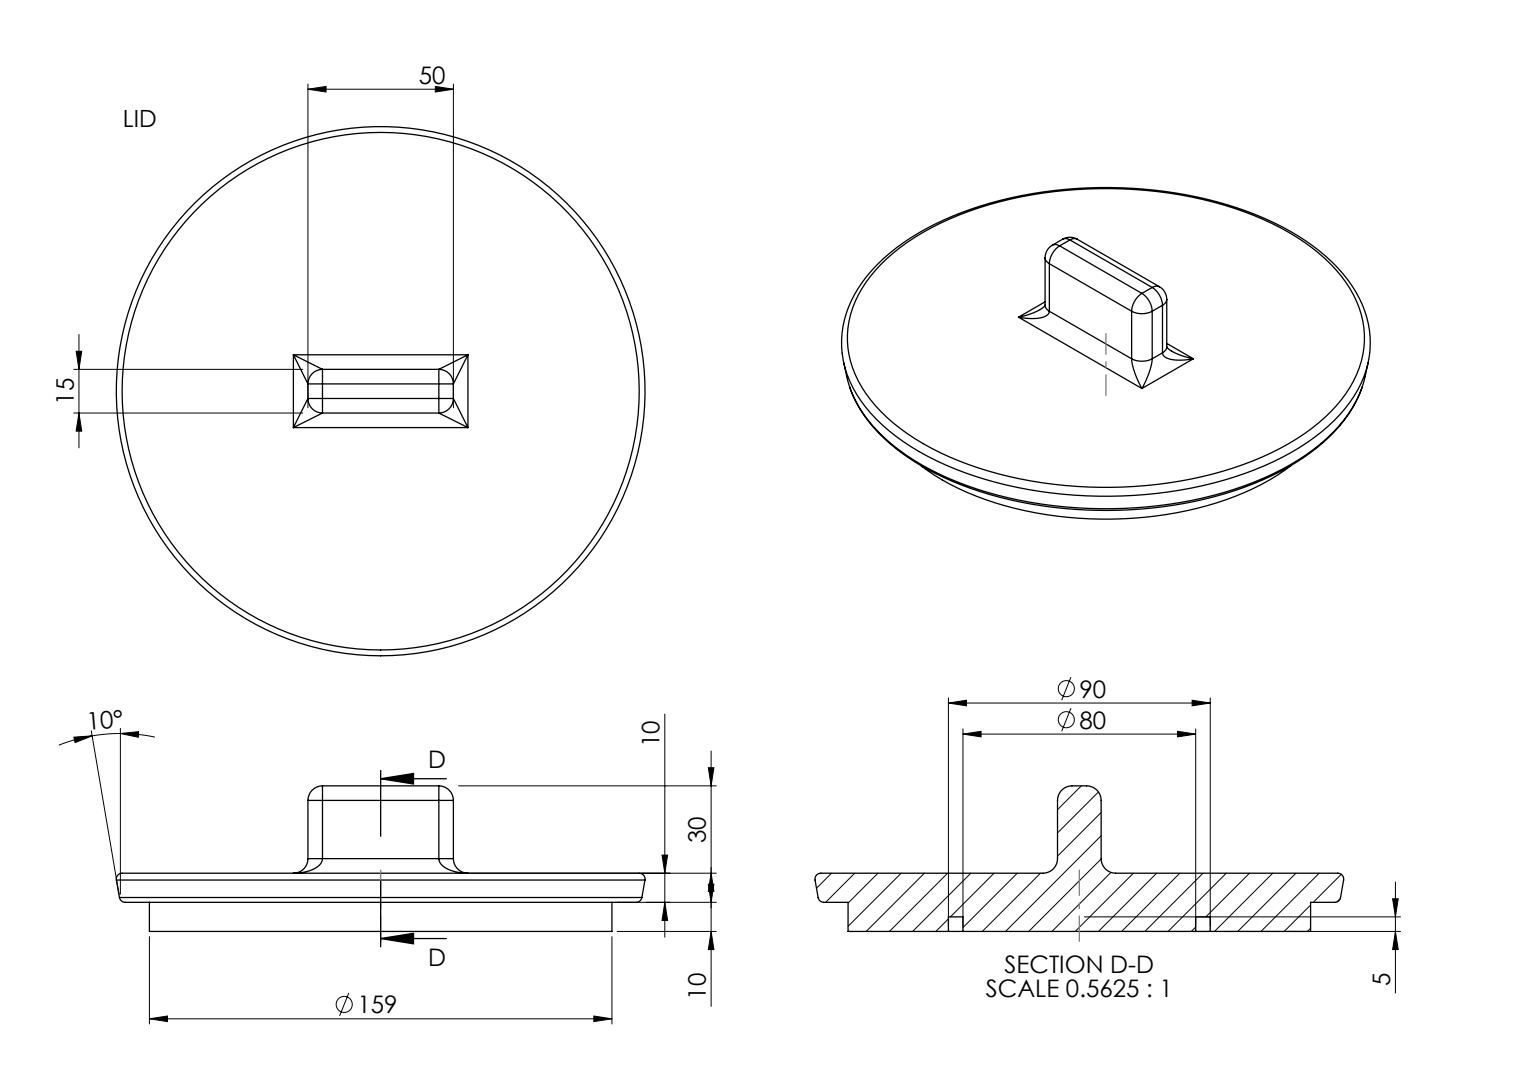
ISO-10303-21;
HEADER;
FILE_DESCRIPTION (('STEP AP214'),
    '1' );
FILE_NAME ('lid.step',
    '2026-10-09T15:02:13',
    ( '' ),
    ( '' ),
    'SwSTEP 2.0',
    'SolidWorks 2026',
    '' );
FILE_SCHEMA (( 'AUTOMOTIVE_DESIGN' ));
ENDSEC;

DATA;
#3=DIRECTION ( 'NONE',  ( 0.000000000000000000, 0.000000000000000000, 1.000000000000000000 ) ) ;
#21=EDGE_LOOP ( 'NONE', ( #2044, #4544 ) ) ;
#25=CARTESIAN_POINT ( 'NONE',  ( 21.01167039530690062, 284.7842439685853719, -8.005835197659997959 ) ) ;
#29=EDGE_CURVE ( 'NONE', #8003, #7684, #9198, .T. ) ;
#39=ORIENTED_EDGE ( 'NONE', *, *, #2245, .T. ) ;
#51=CARTESIAN_POINT ( 'NONE',  ( -30.00000000000000711, 282.0000000000000000, 0.000000000000000000 ) ) ;
#52=ORIENTED_EDGE ( 'NONE', *, *, #15437, .T. ) ;
#55=ORIENTED_EDGE ( 'NONE', *, *, #4586, .T. ) ;
#81=VERTEX_POINT ( 'NONE', #16451 ) ;
#88=CARTESIAN_POINT ( 'NONE',  ( 25.00000000000000000, 284.0710678118655323, -2.499999999999998224 ) ) ;
#98=ORIENTED_EDGE ( 'NONE', *, *, #10995, .T. ) ;
#103=CARTESIAN_POINT ( 'NONE',  ( 28.07127062163609210, 282.3184422169448453, -10.57127062163368691 ) ) ;
#134=AXIS2_PLACEMENT_3D ( 'NONE', #8238, #4509, #8316 ) ;
#139=ORIENTED_EDGE ( 'NONE', *, *, #8040, .T. ) ;
#167=AXIS2_PLACEMENT_3D ( 'NONE', #3146, #15868, #1731 ) ;
#168=AXIS2_PLACEMENT_3D ( 'NONE', #2091, #15059, #8742 ) ;
#190=CARTESIAN_POINT ( 'NONE',  ( 24.98849325795415766, 282.6608420050619088, -9.994246628976295455 ) ) ;
#199=EDGE_CURVE ( 'NONE', #14735, #10689, #4239, .T. ) ;
#223=DIRECTION ( 'NONE',  ( 0.000000000000000000, -1.000000000000000000, 0.000000000000000000 ) ) ;
#233=AXIS2_PLACEMENT_3D ( 'NONE', #3422, #4672, #16139 ) ;
#242=LINE ( 'NONE', #9147, #15465 ) ;
#265=UNCERTAINTY_MEASURE_WITH_UNIT (LENGTH_MEASURE( 1.000000000000000082E-05 ), #1967, 'distance_accuracy_value', 'NONE');
#270=CARTESIAN_POINT ( 'NONE',  ( 26.95005104082769876, 283.0244618719127629, -6.400102081653807673 ) ) ;
#274=CARTESIAN_POINT ( 'NONE',  ( -29.67274705320269135, 282.0000000000000000, 11.84549410641580813 ) ) ;
#302=ORIENTED_EDGE ( 'NONE', *, *, #6524, .T. ) ;
#329=SHAPE_REPRESENTATION ( 'lid', ( #15812 ), #9193 ) ;
#349=ORIENTED_EDGE ( 'NONE', *, *, #7162, .F. ) ;
#353=CARTESIAN_POINT ( 'NONE',  ( 20.51073895446616291, 285.3889217077638705, 7.755369477227151975 ) ) ;
#354=CARTESIAN_POINT ( 'NONE',  ( -27.49424662897630256, 282.6608420050619088, 7.488493257954157656 ) ) ;
#368=CARTESIAN_POINT ( 'NONE',  ( 1.100495818310455813E-14, 282.0000000000000000, -88.87749532708107836 ) ) ;
#381=EDGE_LOOP ( 'NONE', ( #515, #9607 ) ) ;
#395=LINE ( 'NONE', #4248, #7805 ) ;
#429=CIRCLE ( 'NONE', #8137, 79.49773270518484480 ) ;
#443=CARTESIAN_POINT ( 'NONE',  ( -30.00000000000000711, 282.0000000000000000, 12.50000000000000000 ) ) ;
#451=AXIS2_PLACEMENT_3D ( 'NONE', #16347, #7624, #4984 ) ;
#464=PRODUCT_CONTEXT ( 'NONE', #15229, 'mechanical' ) ;
#466=DIRECTION ( 'NONE',  ( 0.000000000000000000, 0.000000000000000000, -1.000000000000000000 ) ) ;
#512=EDGE_CURVE ( 'NONE', #3799, #13515, #6038, .T. ) ;
#515=ORIENTED_EDGE ( 'NONE', *, *, #6228, .F. ) ;
#520=CARTESIAN_POINT ( 'NONE',  ( 22.04892374372132835, 283.9500510409123422, 8.524461871856116701 ) ) ;
#521=CARTESIAN_POINT ( 'NONE',  ( -29.34550962211183744, 282.0322304394514390, 11.19101924422352212 ) ) ;
#581=FACE_BOUND ( 'NONE', #14554, .T. ) ;
#586=AXIS2_PLACEMENT_3D ( 'NONE', #1715, #3134, #466 ) ;
#593=CARTESIAN_POINT ( 'NONE',  ( 28.07127062163604947, 282.3184422169448453, 10.57127062163685949 ) ) ;
#594=CARTESIAN_POINT ( 'NONE',  ( -27.61612561546114009, 282.5087415087664908, 10.11612561546189681 ) ) ;
#621=DIRECTION ( 'NONE',  ( 0.000000000000000000, 0.000000000000000000, 1.000000000000000000 ) ) ;
#630=ADVANCED_FACE ( 'NONE', ( #6188 ), #1425, .F. ) ;
#645=ORIENTED_EDGE ( 'NONE', *, *, #4809, .T. ) ;
#653=DIRECTION ( 'NONE',  ( 0.000000000000000000, 1.000000000000000000, 0.000000000000000000 ) ) ;
#656=AXIS2_PLACEMENT_3D ( 'NONE', #7217, #7053, #1959 ) ;
#675=LINE ( 'NONE', #11094, #3539 ) ;
#676=DIRECTION ( 'NONE',  ( 0.000000000000000000, 0.000000000000000000, -1.000000000000000000 ) ) ;
#714=EDGE_LOOP ( 'NONE', ( #14088, #8765 ) ) ;
#721=CARTESIAN_POINT ( 'NONE',  ( 0.000000000000000000, 272.0000000000000000, 0.000000000000000000 ) ) ;
#728=CARTESIAN_POINT ( 'NONE',  ( 0.000000000000000000, 282.0000000000000000, 0.000000000000000000 ) ) ;
#750=DIRECTION ( 'NONE',  ( 0.000000000000000000, 1.000000000000000000, 0.000000000000000000 ) ) ;
#785=ADVANCED_FACE ( 'NONE', ( #11984 ), #5440, .T. ) ;
#827=DIRECTION ( 'NONE',  ( 1.734723475976807094E-17, 0.000000000000000000, -1.000000000000000000 ) ) ;
#832=EDGE_CURVE ( 'NONE', #2646, #12589, #15834, .T. ) ;
#846=ADVANCED_FACE ( 'NONE', ( #581, #11664 ), #5365, .T. ) ;
#862=ORIENTED_EDGE ( 'NONE', *, *, #15437, .F. ) ;
#870=CARTESIAN_POINT ( 'NONE',  ( -26.23306594130729863, 283.6958662468272792, -4.966131882590582691 ) ) ;
#872=TOROIDAL_SURFACE ( 'NONE', #3283, 88.87749532708107836, 2.000000000000000000 ) ;
#881=LINE ( 'NONE', #9625, #1539 ) ;
#887=CARTESIAN_POINT ( 'NONE',  ( 30.00000000000000000, 282.0000000000000000, 12.50000000000000178 ) ) ;
#891=VERTEX_POINT ( 'NONE', #12993 ) ;
#902=CARTESIAN_POINT ( 'NONE',  ( -2.168404344971008868E-16, 282.0000000000000000, 12.50000000000000000 ) ) ;
#909=CARTESIAN_POINT ( 'NONE',  ( 0.000000000000000000, 262.0000000000000000, 79.49773270518484480 ) ) ;
#944=CARTESIAN_POINT ( 'NONE',  ( 0.000000000000000000, 262.0000000000000000, 0.000000000000000000 ) ) ;
#952=CARTESIAN_POINT ( 'NONE',  ( -24.93825083352641769, 285.3724546740604637, -7.438250833528329942 ) ) ;
#1003=CARTESIAN_POINT ( 'NONE',  ( -25.00000000000000711, 284.0710678118655323, -2.499999999999999556 ) ) ;
#1004=EDGE_LOOP ( 'NONE', ( #10265, #9223, #9244, #3240 ) ) ;
#1036=CARTESIAN_POINT ( 'NONE',  ( -26.95005104082770231, 283.0244618719127629, -6.400102081653810338 ) ) ;
#1039=FACE_OUTER_BOUND ( 'NONE', #9562, .T. ) ;
#1042=VERTEX_POINT ( 'NONE', #14706 ) ;
#1043=DIRECTION ( 'NONE',  ( 0.000000000000000000, 0.000000000000000000, 1.000000000000000000 ) ) ;
#1051=SURFACE_STYLE_USAGE ( .BOTH. , #4992 ) ;
#1066=ORIENTED_EDGE ( 'NONE', *, *, #4920, .T. ) ;
#1070=LINE ( 'NONE', #6161, #12897 ) ;
#1073=DIRECTION ( 'NONE',  ( 0.000000000000000000, 0.000000000000000000, 1.000000000000000000 ) ) ;
#1075=DIRECTION ( 'NONE',  ( -0.000000000000000000, -1.000000000000000000, -0.000000000000000000 ) ) ;
#1106=FACE_OUTER_BOUND ( 'NONE', #13659, .T. ) ;
#1114=CARTESIAN_POINT ( 'NONE',  ( -24.96465690379244862, 286.9981936728224241, -7.464656903793316367 ) ) ;
#1122=CARTESIAN_POINT ( 'NONE',  ( 19.99999999999999289, 307.0000000000000568, -7.500000000000000000 ) ) ;
#1127=( NAMED_UNIT ( * ) SI_UNIT ( $, .STERADIAN. ) SOLID_ANGLE_UNIT ( ) );
#1149=CARTESIAN_POINT ( 'NONE',  ( 25.00000000000000000, 284.0710678118655323, 2.500000000000002220 ) ) ;
#1154=( BOUNDED_CURVE ( )  B_SPLINE_CURVE ( 3, ( #10835, #1003, #11172, #4860 ),
 .UNSPECIFIED., .F., .F. ) 
 B_SPLINE_CURVE_WITH_KNOTS ( ( 4, 4 ),
 ( 3.141592653589793116, 4.712388980384689674 ),
 .UNSPECIFIED. ) 
 CURVE ( )  GEOMETRIC_REPRESENTATION_ITEM ( )  RATIONAL_B_SPLINE_CURVE ( ( 1.000000000000000000, 0.8047378541243649375, 0.8047378541243649375, 1.000000000000000000 ) ) 
 REPRESENTATION_ITEM ( '' )  );
#1171=CARTESIAN_POINT ( 'NONE',  ( 27.07106781186548261, 282.0000000000000000, -6.642135623730952787 ) ) ;
#1184=ORIENTED_EDGE ( 'NONE', *, *, #14174, .T. ) ;
#1197=CARTESIAN_POINT ( 'NONE',  ( -24.86904120090709469, 286.8604097559688739, -7.369041200906229605 ) ) ;
#1209=FACE_OUTER_BOUND ( 'NONE', #12628, .T. ) ;
#1214=EDGE_CURVE ( 'NONE', #8474, #14735, #13959, .T. ) ;
#1223=ORIENTED_EDGE ( 'NONE', *, *, #1722, .F. ) ;
#1226=VERTEX_POINT ( 'NONE', #7814 ) ;
#1247=AXIS2_PLACEMENT_3D ( 'NONE', #12774, #6216, #11211 ) ;
#1255=AXIS2_PLACEMENT_3D ( 'NONE', #8224, #5420, #13290 ) ;
#1277=CARTESIAN_POINT ( 'NONE',  ( 25.50583519765982743, 284.7842439685857698, -3.511670395308112536 ) ) ;
#1303=DIRECTION ( 'NONE',  ( 0.000000000000000000, 0.000000000000000000, 1.000000000000000000 ) ) ;
#1322=DIRECTION ( 'NONE',  ( 0.000000000000000000, -1.000000000000000000, 0.000000000000000000 ) ) ;
#1329=ADVANCED_FACE ( 'NONE', ( #5419 ), #15589, .T. ) ;
#1333=ORIENTED_EDGE ( 'NONE', *, *, #14008, .T. ) ;
#1340=CARTESIAN_POINT ( 'NONE',  ( 25.00000000000000000, 287.0000000000000568, -2.499999999999997780 ) ) ;
#1355=CARTESIAN_POINT ( 'NONE',  ( 23.39173249367926388, 283.2330659412876344, -9.195866246846929215 ) ) ;
#1380=LINE ( 'NONE', #12700, #5056 ) ;
#1402=CARTESIAN_POINT ( 'NONE',  ( 0.000000000000000000, 267.0000000000000000, 0.000000000000000000 ) ) ;
#1409=ORIENTED_EDGE ( 'NONE', *, *, #2371, .T. ) ;
#1410=AXIS2_PLACEMENT_3D ( 'NONE', #16214, #14542, #13953 ) ;
#1417=DIRECTION ( 'NONE',  ( 0.000000000000000000, -1.000000000000000000, 0.000000000000000000 ) ) ;
#1425=CYLINDRICAL_SURFACE ( 'NONE', #14242, 5.000000000000000888 ) ;
#1455=ORIENTED_EDGE ( 'NONE', *, *, #11697, .T. ) ;
#1473=CIRCLE ( 'NONE', #15285, 5.000000000000000000 ) ;
#1486=FACE_OUTER_BOUND ( 'NONE', #4355, .T. ) ;
#1520=CARTESIAN_POINT ( 'NONE',  ( -4.336808689942020818E-17, 307.0000000000000568, 2.500000000000001776 ) ) ;
#1528=CARTESIAN_POINT ( 'NONE',  ( 26.02446187186532001, 283.9500510408986429, -4.548923743720680868 ) ) ;
#1530=DIRECTION ( 'NONE',  ( -1.000000000000000000, -0.000000000000000000, -1.734723475976807094E-17 ) ) ;
#1532=CARTESIAN_POINT ( 'NONE',  ( -26.23306594130729863, 283.6958662468272792, 4.966131882590584468 ) ) ;
#1539=VECTOR ( 'NONE', #7143, 1000.000000000000000 ) ;
#1572=DIRECTION ( 'NONE',  ( 0.000000000000000000, -1.000000000000000000, 0.000000000000000000 ) ) ;
#1580=DIRECTION ( 'NONE',  ( -0.000000000000000000, -1.000000000000000000, -0.000000000000000000 ) ) ;
#1603=( BOUNDED_SURFACE ( )  B_SPLINE_SURFACE ( 3, 2, ( 
 ( #6296, #4813, #7207 ),
 ( #11029, #3384, #2287 ),
 ( #8777, #13760, #10038 ),
 ( #3547, #9866, #14751 ),
 ( #16098, #4732, #7532 ),
 ( #8600, #11365, #8524 ),
 ( #13514, #7379, #12445 ),
 ( #1036, #13839, #12523 ),
 ( #2198, #12268, #7456 ),
 ( #870, #2453, #11204 ),
 ( #7295, #952, #15002 ),
 ( #9790, #11123, #5966 ),
 ( #12603, #12351, #16256 ),
 ( #6053, #4890, #9947 ),
 ( #3638, #1197, #8694 ),
 ( #2373, #1114, #16432 ),
 ( #6210, #11281, #12998 ),
 ( #4101, #11444, #10425 ) ),
 .UNSPECIFIED., .F., .F., .F. ) 
 B_SPLINE_SURFACE_WITH_KNOTS ( ( 4, 2, 2, 2, 2, 2, 2, 2, 4 ),
 ( 3, 3 ),
 ( 1.570796326794896558, 1.767145867644258628, 1.963495408493620697, 2.159844949342982545, 2.356194490192344837, 2.552544031041707129, 2.748893571891068976, 2.945243112740430824, 3.141592653589793116 ),
 ( 0.000000000000000000, 1.000000000000000000 ),
 .UNSPECIFIED. ) 
 GEOMETRIC_REPRESENTATION_ITEM ( )  RATIONAL_B_SPLINE_SURFACE ( (
 ( 1.000000000000000000, 1.000000000000000000, 1.000000000000000000),
 ( 1.000000000000000000, 1.000000000000000000, 1.000000000000000000),
 ( 1.000000000000000000, 0.9967613244521498217, 1.000000000000000000),
 ( 1.000000000000000000, 0.9841171504955907867, 1.000000000000000000),
 ( 1.000000000000000000, 0.9747108043452232806, 1.000000000000000000),
 ( 1.000000000000000000, 0.9506740354170890583, 1.000000000000000000),
 ( 1.000000000000000000, 0.9360421842396997594, 1.000000000000000000),
 ( 1.000000000000000000, 0.9031650994466968729, 1.000000000000000000),
 ( 1.000000000000000000, 0.8849191470854506081, 1.000000000000000000),
 ( 1.000000000000000000, 0.8471316604834270292, 1.000000000000000000),
 ( 1.000000000000000000, 0.8275942695279743244, 1.000000000000000000),
 ( 1.000000000000000000, 0.7902180087153679588, 1.000000000000000000),
 ( 1.000000000000000000, 0.7723968217385259738, 1.000000000000000000),
 ( 1.000000000000000000, 0.7418334179586800747, 1.000000000000000000),
 ( 1.000000000000000000, 0.7291288939600593100, 1.000000000000000000),
 ( 1.000000000000000000, 0.7117460025832584858, 1.000000000000000000),
 ( 1.000000000000000000, 0.7070717283367141670, 1.000000000000000000),
 ( 1.000000000000000000, 0.7071067811865475727, 1.000000000000000000) ) ) 
 REPRESENTATION_ITEM ( '' )  SURFACE ( )  );
#1606=CARTESIAN_POINT ( 'NONE',  ( 21.32168401022778070, 284.4942466289054437, -8.160842005109239850 ) ) ;
#1609=FACE_OUTER_BOUND ( 'NONE', #8042, .T. ) ;
#1610=CARTESIAN_POINT ( 'NONE',  ( -26.77784341583514305, 282.2553694771637538, 10.88892170791705283 ) ) ;
#1613=CARTESIAN_POINT ( 'NONE',  ( 0.000000000000000000, 262.0000000000000000, 0.000000000000000000 ) ) ;
#1689=CARTESIAN_POINT ( 'NONE',  ( 24.96465690379361035, 286.9981936728412393, 7.464656903795364506 ) ) ;
#1691=CARTESIAN_POINT ( 'NONE',  ( -20.31983351293596129, 285.7035871579731179, 7.659916756467385568 ) ) ;
#1715=CARTESIAN_POINT ( 'NONE',  ( 0.000000000000000000, 267.0000000000000000, 0.000000000000000000 ) ) ;
#1722=EDGE_CURVE ( 'NONE', #13617, #14735, #2050, .T. ) ;
#1731=DIRECTION ( 'NONE',  ( 1.224646799147349509E-16, 0.000000000000000000, -1.000000000000000000 ) ) ;
#1748=EDGE_LOOP ( 'NONE', ( #7738, #12625, #11533, #2666 ) ) ;
#1763=AXIS2_PLACEMENT_3D ( 'NONE', #3834, #2583, #12728 ) ;
#1774=CARTESIAN_POINT ( 'NONE',  ( 23.90010208165380590, 283.0244618719131040, 9.450051040827188942 ) ) ;
#1776=CARTESIAN_POINT ( 'NONE',  ( -28.69101924422432148, 282.0322304394514390, 11.84550962211183567 ) ) ;
#1785=AXIS2_PLACEMENT_3D ( 'NONE', #10647, #9394, #14203 ) ;
#1857=EDGE_CURVE ( 'NONE', #3799, #8474, #14802, .T. ) ;
#1923=CARTESIAN_POINT ( 'NONE',  ( 21.32168401022777360, 284.4942466288916307, 8.160842005118437825 ) ) ;
#1933=EDGE_CURVE ( 'NONE', #8272, #81, #7384, .T. ) ;
#1938=ADVANCED_FACE ( 'NONE', ( #16357, #4997 ), #2715, .F. ) ;
#1959=DIRECTION ( 'NONE',  ( 0.000000000000000000, 0.000000000000000000, -1.000000000000000000 ) ) ;
#1967=( LENGTH_UNIT ( ) NAMED_UNIT ( * ) SI_UNIT ( .MILLI., .METRE. ) );
#1985=DIRECTION ( 'NONE',  ( -1.000000000000000000, 0.000000000000000000, -1.734723475976807094E-17 ) ) ;
#2001=AXIS2_PLACEMENT_3D ( 'NONE', #6202, #15242, #4030 ) ;
#2011=CARTESIAN_POINT ( 'NONE',  ( 25.00000000000000000, 287.0000000000000568, 2.500000000000001776 ) ) ;
#2012=CARTESIAN_POINT ( 'NONE',  ( -25.00000000000001066, 287.0000000000000000, 7.500000000000002665 ) ) ;
#2024=EDGE_CURVE ( 'NONE', #10428, #13519, #881, .T. ) ;
#2041=VECTOR ( 'NONE', #1043, 1000.000000000000000 ) ;
#2044=ORIENTED_EDGE ( 'NONE', *, *, #16095, .T. ) ;
#2050=CIRCLE ( 'NONE', #1255, 5.000000000000000000 ) ;
#2052=DIRECTION ( 'NONE',  ( 0.000000000000000000, 1.000000000000000000, 0.000000000000000000 ) ) ;
#2067=ORIENTED_EDGE ( 'NONE', *, *, #5119, .F. ) ;
#2091=CARTESIAN_POINT ( 'NONE',  ( 0.000000000000000000, 267.0000000000000000, 0.000000000000000000 ) ) ;
#2105=EDGE_LOOP ( 'NONE', ( #12917, #9731, #4558, #4173 ) ) ;
#2158=CARTESIAN_POINT ( 'NONE',  ( 0.000000000000000000, 0.000000000000000000, 0.000000000000000000 ) ) ;
#2181=CIRCLE ( 'NONE', #10438, 5.000000000000000000 ) ;
#2183=EDGE_CURVE ( 'NONE', #891, #12043, #14013, .T. ) ;
#2193=CARTESIAN_POINT ( 'NONE',  ( -20.00000000000000355, 307.0000000000000568, -2.499999999999998668 ) ) ;
#2198=CARTESIAN_POINT ( 'NONE',  ( -26.69586624682724718, 283.2330659413073590, -5.891732493678455640 ) ) ;
#2205=ORIENTED_EDGE ( 'NONE', *, *, #199, .F. ) ;
#2232=CARTESIAN_POINT ( 'NONE',  ( 5.510910596163090344E-15, 267.0000000000000000, 45.00000000000000711 ) ) ;
#2237=CARTESIAN_POINT ( 'NONE',  ( -25.00000000000000355, 312.0000000000000568, -7.499999999999999112 ) ) ;
#2244=VECTOR ( 'NONE', #12631, 1000.000000000000000 ) ;
#2245=EDGE_CURVE ( 'NONE', #14735, #12589, #14929, .T. ) ;
#2256=CYLINDRICAL_SURFACE ( 'NONE', #3615, 5.000000000000000000 ) ;
#2287=CARTESIAN_POINT ( 'NONE',  ( -29.34549410641294287, 282.0000000000000000, -12.17274705320727080 ) ) ;
#2296=DIRECTION ( 'NONE',  ( -0.000000000000000000, 1.000000000000000000, 0.000000000000000000 ) ) ;
#2371=EDGE_CURVE ( 'NONE', #13515, #8474, #11913, .T. ) ;
#2373=CARTESIAN_POINT ( 'NONE',  ( -25.03223043950028881, 286.3455096218659151, -2.564460878999442084 ) ) ;
#2378=EDGE_LOOP ( 'NONE', ( #11285, #1066, #14759, #8367 ) ) ;
#2413=LINE ( 'NONE', #11322, #3894 ) ;
#2444=CARTESIAN_POINT ( 'NONE',  ( -27.07106781186547551, 282.0000000000000000, 6.642135623730951899 ) ) ;
#2447=DIRECTION ( 'NONE',  ( 0.000000000000000000, -1.000000000000000000, 0.000000000000000000 ) ) ;
#2453=CARTESIAN_POINT ( 'NONE',  ( -25.07567824489025199, 285.0109613520617131, -7.575678244888824686 ) ) ;
#2462=CARTESIAN_POINT ( 'NONE',  ( -25.00000000000000355, 287.0000000000000568, 7.500000000000001776 ) ) ;
#2464=SURFACE_STYLE_FILL_AREA ( #8872 ) ;
#2466=FILL_AREA_STYLE_COLOUR ( '', #10529 ) ;
#2479=CYLINDRICAL_SURFACE ( 'NONE', #3382, 79.49773270518484480 ) ;
#2520=EDGE_CURVE ( 'NONE', #1226, #4102, #6891, .T. ) ;
#2522=ADVANCED_FACE ( 'NONE', ( #16044 ), #9539, .T. ) ;
#2552=PRESENTATION_STYLE_ASSIGNMENT (( #14019 ) ) ;
#2559=LINE ( 'NONE', #51, #3258 ) ;
#2573=DIRECTION ( 'NONE',  ( -1.000000000000000000, 0.000000000000000000, 0.000000000000000000 ) ) ;
#2577=( BOUNDED_CURVE ( )  B_SPLINE_CURVE ( 3, ( #8071, #11978, #5598, #8162 ),
 .UNSPECIFIED., .F., .F. ) 
 B_SPLINE_CURVE_WITH_KNOTS ( ( 4, 4 ),
 ( 4.712388980384689674, 6.283185307179586232 ),
 .UNSPECIFIED. ) 
 CURVE ( )  GEOMETRIC_REPRESENTATION_ITEM ( )  RATIONAL_B_SPLINE_CURVE ( ( 1.000000000000000000, 0.8047378541243649375, 0.8047378541243649375, 1.000000000000000000 ) ) 
 REPRESENTATION_ITEM ( '' )  );
#2583=DIRECTION ( 'NONE',  ( 0.000000000000000000, 0.000000000000000000, 1.000000000000000000 ) ) ;
#2584=ADVANCED_FACE ( 'NONE', ( #3671 ), #6491, .T. ) ;
#2602=ADVANCED_FACE ( 'NONE', ( #5264 ), #7653, .T. ) ;
#2612=CARTESIAN_POINT ( 'NONE',  ( 25.75618375337248978, 283.9316295015381115, -8.256183753373985468 ) ) ;
#2616=CYLINDRICAL_SURFACE ( 'NONE', #15808, 5.000000000000000000 ) ;
#2635=( GEOMETRIC_REPRESENTATION_CONTEXT ( 3 ) GLOBAL_UNCERTAINTY_ASSIGNED_CONTEXT ( ( #12754 ) ) GLOBAL_UNIT_ASSIGNED_CONTEXT ( ( #15017, #15102, #1127 ) ) REPRESENTATION_CONTEXT ( 'NONE', 'WORKASPACE' ) );
#2636=( NAMED_UNIT ( * ) SI_UNIT ( $, .STERADIAN. ) SOLID_ANGLE_UNIT ( ) );
#2646=VERTEX_POINT ( 'NONE', #9064 ) ;
#2666=ORIENTED_EDGE ( 'NONE', *, *, #4217, .F. ) ;
#2689=CARTESIAN_POINT ( 'NONE',  ( 25.66084200510924518, 284.4942466289054437, -3.821684010228425077 ) ) ;
#2693=DIRECTION ( 'NONE',  ( 0.000000000000000000, -0.000000000000000000, 1.000000000000000000 ) ) ;
#2715=PLANE ( 'NONE',  #8699 ) ;
#2751=FACE_OUTER_BOUND ( 'NONE', #7948, .T. ) ;
#2759=DIRECTION ( 'NONE',  ( 1.734723475976807094E-17, 0.000000000000000000, -1.000000000000000000 ) ) ;
#2760=AXIS2_PLACEMENT_3D ( 'NONE', #1402, #1075, #7654 ) ;
#2770=CARTESIAN_POINT ( 'NONE',  ( 26.40559293885987557, 283.2826504366940412, -8.905592938858417185 ) ) ;
#2776=CARTESIAN_POINT ( 'NONE',  ( -23.39173249367811636, 283.2330659413077001, 9.195866246826893686 ) ) ;
#2787=ORIENTED_EDGE ( 'NONE', *, *, #12706, .F. ) ;
#2790=DIRECTION ( 'NONE',  ( -1.000000000000000000, 0.000000000000000000, -2.602085213965210149E-16 ) ) ;
#2807=ORIENTED_EDGE ( 'NONE', *, *, #10077, .T. ) ;
#2812=AXIS2_PLACEMENT_3D ( 'NONE', #8014, #12076, #15734 ) ;
#2851=DIRECTION ( 'NONE',  ( 0.000000000000000000, 0.000000000000000000, -1.000000000000000000 ) ) ;
#2860=CARTESIAN_POINT ( 'NONE',  ( 29.67274705320743777, 282.0000000000000000, -11.84549410641326084 ) ) ;
#2866=FACE_OUTER_BOUND ( 'NONE', #2972, .T. ) ;
#2905=VECTOR ( 'NONE', #3482, 1000.000000000000000 ) ;
#2909=CARTESIAN_POINT ( 'NONE',  ( 0.000000000000000000, 312.0000000000000568, 0.000000000000000000 ) ) ;
#2915=DIRECTION ( 'NONE',  ( -0.000000000000000000, 1.000000000000000000, -0.000000000000000000 ) ) ;
#2925=PLANE ( 'NONE',  #10258 ) ;
#2932=CARTESIAN_POINT ( 'NONE',  ( 19.99999999999999645, 287.0000000000000568, 2.500000000000002220 ) ) ;
#2943=CARTESIAN_POINT ( 'NONE',  ( 28.70358715772642455, 282.1599167565164521, 9.907174315453913138 ) ) ;
#2944=CARTESIAN_POINT ( 'NONE',  ( -25.50583519766042429, 284.7842439685843487, 3.511670395308091219 ) ) ;
#2956=ORIENTED_EDGE ( 'NONE', *, *, #12706, .T. ) ;
#2972=EDGE_LOOP ( 'NONE', ( #15403, #2205, #1223 ) ) ;
#2973=CARTESIAN_POINT ( 'NONE',  ( -30.00000000000000711, 282.0000000000000000, 12.50000000000000000 ) ) ;
#2988=VECTOR ( 'NONE', #14774, 1000.000000000000000 ) ;
#2998=AXIS2_PLACEMENT_3D ( 'NONE', #6852, #13232, #9408 ) ;
#3005=CARTESIAN_POINT ( 'NONE',  ( -20.00000000000000355, 307.0000000000000568, -2.499999999999998668 ) ) ;
#3011=AXIS2_PLACEMENT_3D ( 'NONE', #3005, #14221, #6857 ) ;
#3019=CARTESIAN_POINT ( 'NONE',  ( 25.75618375337400678, 283.9316295015381115, 8.256183753372502210 ) ) ;
#3021=CARTESIAN_POINT ( 'NONE',  ( -27.40717431545314042, 282.1599167565163384, 11.20358715772689528 ) ) ;
#3034=ORIENTED_EDGE ( 'NONE', *, *, #9677, .T. ) ;
#3049=ORIENTED_EDGE ( 'NONE', *, *, #3118, .T. ) ;
#3066=CIRCLE ( 'NONE', #12357, 90.84711083310548929 ) ;
#3077=CIRCLE ( 'NONE', #14231, 5.000000000000000888 ) ;
#3093=EDGE_CURVE ( 'NONE', #9838, #13826, #12732, .T. ) ;
#3094=AXIS2_PLACEMENT_3D ( 'NONE', #1520, #9414, #2759 ) ;
#3097=AXIS2_PLACEMENT_3D ( 'NONE', #10227, #3826, #2573 ) ;
#3106=CARTESIAN_POINT ( 'NONE',  ( 27.61612561545807409, 282.5087415087664908, 10.11612561546265354 ) ) ;
#3107=EDGE_CURVE ( 'NONE', #3799, #1042, #12368, .T. ) ;
#3108=AXIS2_PLACEMENT_3D ( 'NONE', #15384, #10159, #8234 ) ;
#3109=CARTESIAN_POINT ( 'NONE',  ( -20.06446087899944786, 286.3455096218657445, 7.532230439500318120 ) ) ;
#3118=EDGE_CURVE ( 'NONE', #12043, #12621, #13851, .T. ) ;
#3121=EDGE_LOOP ( 'NONE', ( #4200, #5539, #1333, #14827 ) ) ;
#3126=CARTESIAN_POINT ( 'NONE',  ( -20.00000000000000355, 307.0000000000000568, -2.499999999999998668 ) ) ;
#3134=DIRECTION ( 'NONE',  ( 0.000000000000000000, -1.000000000000000000, 0.000000000000000000 ) ) ;
#3146=CARTESIAN_POINT ( 'NONE',  ( 1.075479105333760460E-14, 274.0000000000000000, -87.81953344283027718 ) ) ;
#3159=EDGE_CURVE ( 'NONE', #7881, #2646, #1380, .T. ) ;
#3172=ADVANCED_FACE ( 'NONE', ( #15260 ), #3969, .F. ) ;
#3187=MANIFOLD_SOLID_BREP ( 'Cut-Extrude1', #7606 ) ;
#3190=FACE_OUTER_BOUND ( 'NONE', #15995, .T. ) ;
#3201=VERTEX_POINT ( 'NONE', #3889 ) ;
#3203=DIRECTION ( 'NONE',  ( 0.000000000000000000, 1.000000000000000000, 0.000000000000000000 ) ) ;
#3218=FACE_OUTER_BOUND ( 'NONE', #10834, .T. ) ;
#3240=ORIENTED_EDGE ( 'NONE', *, *, #6712, .F. ) ;
#3245=CARTESIAN_POINT ( 'NONE',  ( 0.000000000000000000, 267.0000000000000000, 0.000000000000000000 ) ) ;
#3258=VECTOR ( 'NONE', #5156, 1000.000000000000000 ) ;
#3266=CARTESIAN_POINT ( 'NONE',  ( 24.99999999999999645, 312.0000000000000568, 7.500000000000002665 ) ) ;
#3268=CARTESIAN_POINT ( 'NONE',  ( -25.00000000000000711, 287.0000000000000568, 2.500000000000002220 ) ) ;
#3283=AXIS2_PLACEMENT_3D ( 'NONE', #5171, #7564, #11469 ) ;
#3288=DIRECTION ( 'NONE',  ( -0.000000000000000000, 1.000000000000000000, 0.000000000000000000 ) ) ;
#3301=CARTESIAN_POINT ( 'NONE',  ( 0.000000000000000000, 273.6527036446661896, 0.000000000000000000 ) ) ;
#3326=LINE ( 'NONE', #902, #8216 ) ;
#3333=CARTESIAN_POINT ( 'NONE',  ( -20.00000000000000711, 284.0710678118654755, -7.499999999999999112 ) ) ;
#3346=STYLED_ITEM ( 'NONE', ( #2552 ), #7430 ) ;
#3363=EDGE_CURVE ( 'NONE', #7238, #10689, #3326, .T. ) ;
#3382=AXIS2_PLACEMENT_3D ( 'NONE', #15114, #7559, #8719 ) ;
#3384=CARTESIAN_POINT ( 'NONE',  ( -29.50911996093393341, 282.0000000000000000, -12.00911996094034961 ) ) ;
#3411=ORIENTED_EDGE ( 'NONE', *, *, #8538, .T. ) ;
#3422=CARTESIAN_POINT ( 'NONE',  ( 0.000000000000000000, 272.0000000000000000, 0.000000000000000000 ) ) ;
#3482=DIRECTION ( 'NONE',  ( -0.000000000000000000, -0.000000000000000000, -1.000000000000000000 ) ) ;
#3484=( NAMED_UNIT ( * ) PLANE_ANGLE_UNIT ( ) SI_UNIT ( $, .RADIAN. ) );
#3503=FACE_OUTER_BOUND ( 'NONE', #5085, .T. ) ;
#3504=CARTESIAN_POINT ( 'NONE',  ( -20.00000000000000355, 307.0000000000000568, 2.500000000000001332 ) ) ;
#3539=VECTOR ( 'NONE', #5938, 1000.000000000000000 ) ;
#3542=SPHERICAL_SURFACE ( 'NONE', #8622, 5.000000000000000000 ) ;
#3547=CARTESIAN_POINT ( 'NONE',  ( -28.70358715772690061, 282.1599167565163384, -9.907174315453927349 ) ) ;
#3552=ORIENTED_EDGE ( 'NONE', *, *, #8040, .F. ) ;
#3553=ORIENTED_EDGE ( 'NONE', *, *, #8956, .T. ) ;
#3555=EDGE_CURVE ( 'NONE', #11555, #891, #8750, .T. ) ;
#3559=DIRECTION ( 'NONE',  ( 1.000000000000000000, -0.000000000000000000, 1.734723475976807094E-17 ) ) ;
#3573=EDGE_LOOP ( 'NONE', ( #7136, #645, #15857, #5332 ) ) ;
#3580=FACE_OUTER_BOUND ( 'NONE', #5253, .T. ) ;
#3602=DIRECTION ( 'NONE',  ( -0.000000000000000000, -1.000000000000000000, -0.000000000000000000 ) ) ;
#3615=AXIS2_PLACEMENT_3D ( 'NONE', #5188, #1417, #5035 ) ;
#3624=VECTOR ( 'NONE', #15715, 1000.000000000000000 ) ;
#3627=CIRCLE ( 'NONE', #16086, 5.000000000000000888 ) ;
#3638=CARTESIAN_POINT ( 'NONE',  ( -25.15991675646742465, 285.7035871579729474, -2.819833512935953301 ) ) ;
#3652=AXIS2_PLACEMENT_3D ( 'NONE', #3266, #5388, #15424 ) ;
#3663=FACE_OUTER_BOUND ( 'NONE', #12089, .T. ) ;
#3671=FACE_OUTER_BOUND ( 'NONE', #3573, .T. ) ;
#3685=VECTOR ( 'NONE', #3559, 1000.000000000000000 ) ;
#3709=VECTOR ( 'NONE', #6145, 1000.000000000000000 ) ;
#3713=DIRECTION ( 'NONE',  ( 0.000000000000000000, 0.000000000000000000, -1.000000000000000000 ) ) ;
#3731=DIRECTION ( 'NONE',  ( 0.000000000000000000, 1.000000000000000000, 0.000000000000000000 ) ) ;
#3733=ORIENTED_EDGE ( 'NONE', *, *, #5119, .T. ) ;
#3735=ORIENTED_EDGE ( 'NONE', *, *, #4217, .T. ) ;
#3749=CARTESIAN_POINT ( 'NONE',  ( 25.00000000000000000, 287.0000000000000568, -2.499999999999997780 ) ) ;
#3761=CARTESIAN_POINT ( 'NONE',  ( 0.000000000000000000, 282.0000000000000000, 0.000000000000000000 ) ) ;
#3783=CARTESIAN_POINT ( 'NONE',  ( 20.06446087900059894, 286.3455096218831386, -7.532230439496852448 ) ) ;
#3799=VERTEX_POINT ( 'NONE', #9307 ) ;
#3800=VECTOR ( 'NONE', #5369, 1000.000000000000000 ) ;
#3814=ORIENTED_EDGE ( 'NONE', *, *, #3363, .F. ) ;
#3826=DIRECTION ( 'NONE',  ( 0.000000000000000000, 1.000000000000000000, 0.000000000000000000 ) ) ;
#3834=CARTESIAN_POINT ( 'NONE',  ( -20.00000000000000355, 307.0000000000000568, 0.000000000000000000 ) ) ;
#3863=CARTESIAN_POINT ( 'NONE',  ( 30.00000000000000711, 282.0000000000000000, -12.50000000000000000 ) ) ;
#3889=CARTESIAN_POINT ( 'NONE',  ( 0.000000000000000000, 273.6527036446661896, 89.78914894885470233 ) ) ;
#3894=VECTOR ( 'NONE', #5023, 1000.000000000000000 ) ;
#3906=CARTESIAN_POINT ( 'NONE',  ( 30.00000000000000355, 282.0000000000000000, 6.938893903907227589E-15 ) ) ;
#3914=CARTESIAN_POINT ( 'NONE',  ( 0.000000000000000000, 279.6527036446661327, 90.84711083310548929 ) ) ;
#3919=ORIENTED_EDGE ( 'NONE', *, *, #3118, .F. ) ;
#3945=CARTESIAN_POINT ( 'NONE',  ( 25.48725218877856946, 284.2907069533056301, -7.987252188780951556 ) ) ;
#3949=FACE_OUTER_BOUND ( 'NONE', #14803, .T. ) ;
#3963=LINE ( 'NONE', #6387, #14456 ) ;
#3969=CYLINDRICAL_SURFACE ( 'NONE', #11673, 5.000000000000000888 ) ;
#3974=CARTESIAN_POINT ( 'NONE',  ( 0.000000000000000000, 272.0000000000000000, 0.000000000000000000 ) ) ;
#3992=DIRECTION ( 'NONE',  ( 0.000000000000000000, 0.000000000000000000, -1.000000000000000000 ) ) ;
#4018=DIRECTION ( 'NONE',  ( 1.000000000000000000, 0.000000000000000000, 0.000000000000000000 ) ) ;
#4026=CARTESIAN_POINT ( 'NONE',  ( 24.81239020281854835, 286.7275190727439735, -7.312390202817915075 ) ) ;
#4030=DIRECTION ( 'NONE',  ( -1.000000000000000000, 0.000000000000000000, 0.000000000000000000 ) ) ;
#4101=CARTESIAN_POINT ( 'NONE',  ( -25.00000000000000711, 287.0000000000000568, -2.500000000000000444 ) ) ;
#4102=VERTEX_POINT ( 'NONE', #7542 ) ;
#4108=CARTESIAN_POINT ( 'NONE',  ( 24.93825083353323535, 285.3724546740180017, -7.438250833534492124 ) ) ;
#4112=CARTESIAN_POINT ( 'NONE',  ( 28.38892170791706349, 282.2553694771637538, 9.277843415834380991 ) ) ;
#4114=CARTESIAN_POINT ( 'NONE',  ( -28.07127062163743503, 282.3184422169439927, 10.57127062163423759 ) ) ;
#4155=DIRECTION ( 'NONE',  ( 1.000000000000000000, 0.000000000000000000, 1.734723475976807094E-17 ) ) ;
#4173=ORIENTED_EDGE ( 'NONE', *, *, #9270, .T. ) ;
#4181=ORIENTED_EDGE ( 'NONE', *, *, #1933, .T. ) ;
#4182=DIRECTION ( 'NONE',  ( 0.000000000000000000, -1.000000000000000000, 0.000000000000000000 ) ) ;
#4200=ORIENTED_EDGE ( 'NONE', *, *, #10371, .F. ) ;
#4205=CARTESIAN_POINT ( 'NONE',  ( 24.86904120090595072, 286.8604097559505703, 7.369041200904230315 ) ) ;
#4217=EDGE_CURVE ( 'NONE', #15703, #3201, #11579, .T. ) ;
#4235=CARTESIAN_POINT ( 'NONE',  ( -24.14213562373094746, 282.0000000000000000, 9.571067811865473729 ) ) ;
#4238=CARTESIAN_POINT ( 'NONE',  ( -4.336808689942020818E-17, 312.0000000000000568, 2.500000000000001776 ) ) ;
#4239=( BOUNDED_CURVE ( )  B_SPLINE_CURVE ( 3, ( #10556, #9303, #4235, #2973 ),
 .UNSPECIFIED., .F., .T. ) 
 B_SPLINE_CURVE_WITH_KNOTS ( ( 4, 4 ),
 ( 3.141592653589793116, 4.712388980384689674 ),
 .UNSPECIFIED. ) 
 CURVE ( )  GEOMETRIC_REPRESENTATION_ITEM ( )  RATIONAL_B_SPLINE_CURVE ( ( 1.000000000000000000, 0.8047378541243649375, 0.8047378541243649375, 1.000000000000000000 ) ) 
 REPRESENTATION_ITEM ( '' )  );
#4248=CARTESIAN_POINT ( 'NONE',  ( 19.99999999999999289, 312.0000000000000568, -7.500000000000000000 ) ) ;
#4252=CARTESIAN_POINT ( 'NONE',  ( 5.510910596163090344E-15, 267.0000000000000000, 45.00000000000000711 ) ) ;
#4277=ORIENTED_EDGE ( 'NONE', *, *, #5509, .T. ) ;
#4279=PRODUCT_DEFINITION ( 'UNKNOWN', '', #15287, #5292 ) ;
#4284=CARTESIAN_POINT ( 'NONE',  ( -25.03223043950028881, 286.3455096218659151, 2.564460878999443860 ) ) ;
#4333=ORIENTED_EDGE ( 'NONE', *, *, #3107, .T. ) ;
#4341=CARTESIAN_POINT ( 'NONE',  ( 19.99999999999999645, 312.0000000000000568, 2.500000000000002220 ) ) ;
#4353=AXIS2_PLACEMENT_3D ( 'NONE', #16293, #4929, #9984 ) ;
#4355=EDGE_LOOP ( 'NONE', ( #15233, #14760, #6174 ) ) ;
#4360=CARTESIAN_POINT ( 'NONE',  ( 25.50583519765999796, 284.7842439685853719, 3.511670395308114312 ) ) ;
#4362=CARTESIAN_POINT ( 'NONE',  ( -24.78235906513968345, 286.0218276481963358, 7.282359065138694909 ) ) ;
#4375=VERTEX_POINT ( 'NONE', #8518 ) ;
#4378=EDGE_CURVE ( 'NONE', #16375, #9704, #4416, .T. ) ;
#4411=EDGE_LOOP ( 'NONE', ( #13539, #5003 ) ) ;
#4416=CIRCLE ( 'NONE', #7060, 79.49773270518484480 ) ;
#4451=CARTESIAN_POINT ( 'NONE',  ( -25.66084200511936686, 284.4942466288902096, 3.821684010227676342 ) ) ;
#4490=AXIS2_PLACEMENT_3D ( 'NONE', #12722, #11547, #3992 ) ;
#4508=FACE_OUTER_BOUND ( 'NONE', #5232, .T. ) ;
#4509=DIRECTION ( 'NONE',  ( 2.312964634635742464E-16, 0.000000000000000000, -1.000000000000000000 ) ) ;
#4513=ADVANCED_FACE ( 'NONE', ( #1106 ), #13999, .T. ) ;
#4529=CARTESIAN_POINT ( 'NONE',  ( 24.99999979512263693, 287.0011899277170073, 7.499999795122639590 ) ) ;
#4544=ORIENTED_EDGE ( 'NONE', *, *, #14807, .T. ) ;
#4558=ORIENTED_EDGE ( 'NONE', *, *, #12595, .T. ) ;
#4586=EDGE_CURVE ( 'NONE', #10689, #13617, #5409, .T. ) ;
#4592=ADVANCED_FACE ( 'NONE', ( #3949 ), #2616, .F. ) ;
#4599=CONICAL_SURFACE ( 'NONE', #11745, 89.49773270518483059, 0.1745329251994333364 ) ;
#4611=DIRECTION ( 'NONE',  ( 0.000000000000000000, 1.000000000000000000, 0.000000000000000000 ) ) ;
#4618=ADVANCED_FACE ( 'NONE', ( #10031, #12594 ), #15330, .F. ) ;
#4625=ORIENTED_EDGE ( 'NONE', *, *, #9567, .T. ) ;
#4642=ORIENTED_EDGE ( 'NONE', *, *, #9388, .F. ) ;
#4646=VECTOR ( 'NONE', #1530, 1000.000000000000000 ) ;
#4660=EDGE_LOOP ( 'NONE', ( #12509, #4277, #12222, #12384 ) ) ;
#4671=DIRECTION ( 'NONE',  ( -0.000000000000000000, -1.000000000000000000, -0.000000000000000000 ) ) ;
#4672=DIRECTION ( 'NONE',  ( 0.000000000000000000, 1.000000000000000000, 0.000000000000000000 ) ) ;
#4707=ADVANCED_FACE ( 'NONE', ( #2866 ), #10503, .T. ) ;
#4710=ORIENTED_EDGE ( 'NONE', *, *, #12618, .F. ) ;
#4712=VERTEX_POINT ( 'NONE', #11003 ) ;
#4732=CARTESIAN_POINT ( 'NONE',  ( -27.61612561546114009, 282.5087415087664908, -10.11612561546113298 ) ) ;
#4755=DIRECTION ( 'NONE',  ( 0.000000000000000000, 0.000000000000000000, -1.000000000000000000 ) ) ;
#4766=FACE_OUTER_BOUND ( 'NONE', #12852, .T. ) ;
#4770=CARTESIAN_POINT ( 'NONE',  ( 0.000000000000000000, 274.0000000000000000, 0.000000000000000000 ) ) ;
#4797=EDGE_CURVE ( 'NONE', #2646, #7011, #11180, .T. ) ;
#4800=AXIS2_PLACEMENT_3D ( 'NONE', #7481, #5168, #11466 ) ;
#4809=EDGE_CURVE ( 'NONE', #11650, #4712, #12105, .T. ) ;
#4813=CARTESIAN_POINT ( 'NONE',  ( -30.00000000000000711, 282.0000000000000000, -12.49999999999999822 ) ) ;
#4850=DIRECTION ( 'NONE',  ( 0.000000000000000000, 0.000000000000000000, 1.000000000000000000 ) ) ;
#4860=CARTESIAN_POINT ( 'NONE',  ( -30.00000000000000711, 282.0000000000000000, -12.49999999999999822 ) ) ;
#4890=CARTESIAN_POINT ( 'NONE',  ( -24.81239020281865137, 286.7275190727449967, -7.312390202818956908 ) ) ;
#4898=CARTESIAN_POINT ( 'NONE',  ( 0.000000000000000000, 262.0000000000000000, 79.49773270518484480 ) ) ;
#4903=AXIS2_PLACEMENT_3D ( 'NONE', #4770, #12059, #4850 ) ;
#4917=ORIENTED_EDGE ( 'NONE', *, *, #11691, .F. ) ;
#4920=EDGE_CURVE ( 'NONE', #13519, #7011, #12188, .T. ) ;
#4929=DIRECTION ( 'NONE',  ( 1.000000000000000000, 0.000000000000000000, 0.000000000000000000 ) ) ;
#4930=DIRECTION ( 'NONE',  ( -0.000000000000000000, -1.000000000000000000, -0.000000000000000000 ) ) ;
#4979=CIRCLE ( 'NONE', #167, 2.000000000000001776 ) ;
#4984=DIRECTION ( 'NONE',  ( 0.000000000000000000, 0.000000000000000000, -1.000000000000000000 ) ) ;
#4985=CYLINDRICAL_SURFACE ( 'NONE', #8099, 5.000000000000000888 ) ;
#4986=EDGE_CURVE ( 'NONE', #4102, #1226, #429, .T. ) ;
#4992=SURFACE_SIDE_STYLE ('',( #2464 ) ) ;
#4993=AXIS2_PLACEMENT_3D ( 'NONE', #3301, #2052, #11038 ) ;
#4997=FACE_BOUND ( 'NONE', #4411, .T. ) ;
#5003=ORIENTED_EDGE ( 'NONE', *, *, #4986, .T. ) ;
#5006=VERTEX_POINT ( 'NONE', #5037 ) ;
#5023=DIRECTION ( 'NONE',  ( -0.000000000000000000, -1.000000000000000000, -0.000000000000000000 ) ) ;
#5030=ORIENTED_EDGE ( 'NONE', *, *, #5371, .T. ) ;
#5035=DIRECTION ( 'NONE',  ( 0.000000000000000000, 0.000000000000000000, -1.000000000000000000 ) ) ;
#5037=CARTESIAN_POINT ( 'NONE',  ( 5.510910596163090344E-15, 262.0000000000000000, 45.00000000000000711 ) ) ;
#5054=CARTESIAN_POINT ( 'NONE',  ( 19.99999999999659650, 286.6727470533784867, -7.500000000000000888 ) ) ;
#5056=VECTOR ( 'NONE', #10048, 1000.000000000000000 ) ;
#5057=DIRECTION ( 'NONE',  ( 0.000000000000000000, -1.000000000000000000, 0.000000000000000000 ) ) ;
#5061=CARTESIAN_POINT ( 'NONE',  ( 0.000000000000000000, 262.0000000000000000, 0.000000000000000000 ) ) ;
#5075=DIRECTION ( 'NONE',  ( 2.312964634635742464E-16, 0.000000000000000000, -1.000000000000000000 ) ) ;
#5085=EDGE_LOOP ( 'NONE', ( #6765, #15836, #3049, #13778 ) ) ;
#5115=LINE ( 'NONE', #14062, #9212 ) ;
#5119=EDGE_CURVE ( 'NONE', #1042, #11555, #10663, .T. ) ;
#5131=CARTESIAN_POINT ( 'NONE',  ( 28.70358715772643166, 282.1599167565164521, -9.907174315453913138 ) ) ;
#5156=DIRECTION ( 'NONE',  ( -0.000000000000000000, -0.000000000000000000, -1.000000000000000000 ) ) ;
#5168=DIRECTION ( 'NONE',  ( -0.000000000000000000, -1.000000000000000000, -0.000000000000000000 ) ) ;
#5171=CARTESIAN_POINT ( 'NONE',  ( 0.000000000000000000, 280.0000000000000000, 0.000000000000000000 ) ) ;
#5188=CARTESIAN_POINT ( 'NONE',  ( 19.99999999999999289, 312.0000000000000568, -2.499999999999999556 ) ) ;
#5208=CARTESIAN_POINT ( 'NONE',  ( 28.69101924422354699, 282.0322304394513253, -11.84550962211230107 ) ) ;
#5213=CARTESIAN_POINT ( 'NONE',  ( -25.00000000000000711, 284.0710678118654755, 2.500000000000003109 ) ) ;
#5232=EDGE_LOOP ( 'NONE', ( #12679, #15207, #10306, #12693 ) ) ;
#5233=( GEOMETRIC_REPRESENTATION_CONTEXT ( 3 ) GLOBAL_UNCERTAINTY_ASSIGNED_CONTEXT ( ( #15231 ) ) GLOBAL_UNIT_ASSIGNED_CONTEXT ( ( #14936, #15104, #13933 ) ) REPRESENTATION_CONTEXT ( 'NONE', 'WORKASPACE' ) );
#5253=EDGE_LOOP ( 'NONE', ( #39, #14838, #139, #10062 ) ) ;
#5264=FACE_OUTER_BOUND ( 'NONE', #9375, .T. ) ;
#5275=CARTESIAN_POINT ( 'NONE',  ( -25.00000000000000355, 287.0000000000000568, -2.499999999999998668 ) ) ;
#5292=PRODUCT_DEFINITION_CONTEXT ( 'detailed design', #13231, 'design' ) ;
#5297=CARTESIAN_POINT ( 'NONE',  ( 28.38892170791706704, 282.2553694771637538, -9.277843415834380991 ) ) ;
#5332=ORIENTED_EDGE ( 'NONE', *, *, #29, .F. ) ;
#5365=PLANE ( 'NONE',  #9224 ) ;
#5369=DIRECTION ( 'NONE',  ( -0.000000000000000000, 1.000000000000000000, -0.000000000000000000 ) ) ;
#5371=EDGE_CURVE ( 'NONE', #11650, #8003, #6093, .T. ) ;
#5375=CARTESIAN_POINT ( 'NONE',  ( 27.61612561545959821, 282.5087415087664340, -10.11612561546112943 ) ) ;
#5378=CARTESIAN_POINT ( 'NONE',  ( -26.02446187185519832, 283.9500510409137632, 4.548923743721434043 ) ) ;
#5388=DIRECTION ( 'NONE',  ( -1.000000000000000000, 0.000000000000000000, -2.312964634635742464E-16 ) ) ;
#5393=DIRECTION ( 'NONE',  ( -0.000000000000000000, -1.000000000000000000, -0.000000000000000000 ) ) ;
#5400=EDGE_CURVE ( 'NONE', #7011, #13460, #16112, .T. ) ;
#5409=( BOUNDED_CURVE ( )  B_SPLINE_CURVE ( 3, ( #11511, #2444, #5213, #12762 ),
 .UNSPECIFIED., .F., .T. ) 
 B_SPLINE_CURVE_WITH_KNOTS ( ( 4, 4 ),
 ( 1.570796326794896780, 3.141592653589793116 ),
 .UNSPECIFIED. ) 
 CURVE ( )  GEOMETRIC_REPRESENTATION_ITEM ( )  RATIONAL_B_SPLINE_CURVE ( ( 1.000000000000000000, 0.8047378541243650485, 0.8047378541243650485, 1.000000000000000000 ) ) 
 REPRESENTATION_ITEM ( '' )  );
#5419=FACE_OUTER_BOUND ( 'NONE', #10691, .T. ) ;
#5420=DIRECTION ( 'NONE',  ( 0.000000000000000000, 1.000000000000000000, -0.000000000000000000 ) ) ;
#5440=CYLINDRICAL_SURFACE ( 'NONE', #3094, 5.000000000000000000 ) ;
#5453=CARTESIAN_POINT ( 'NONE',  ( 26.23306594128796121, 283.6958662468466059, 4.966131882590526736 ) ) ;
#5454=CARTESIAN_POINT ( 'NONE',  ( -22.46613188259093974, 283.6958662468269949, 8.733065941307639690 ) ) ;
#5463=VECTOR ( 'NONE', #12791, 1000.000000000000000 ) ;
#5508=CYLINDRICAL_SURFACE ( 'NONE', #13598, 5.000000000000000000 ) ;
#5509=EDGE_CURVE ( 'NONE', #8227, #1042, #3627, .T. ) ;
#5539=ORIENTED_EDGE ( 'NONE', *, *, #9567, .F. ) ;
#5544=CARTESIAN_POINT ( 'NONE',  ( -24.96465690379244862, 286.9981936728224241, 7.464656903793317255 ) ) ;
#5558=DIRECTION ( 'NONE',  ( -0.000000000000000000, -1.000000000000000000, -0.000000000000000000 ) ) ;
#5598=CARTESIAN_POINT ( 'NONE',  ( 20.00000000000000355, 284.0710678118655323, 7.500000000000000000 ) ) ;
#5603=DIRECTION ( 'NONE',  ( 0.000000000000000000, -1.000000000000000000, 0.000000000000000000 ) ) ;
#5613=CARTESIAN_POINT ( 'NONE',  ( 24.98849325795415055, 282.6608420050615678, 9.994246628976808822 ) ) ;
#5616=CARTESIAN_POINT ( 'NONE',  ( -26.69586624682724718, 283.2330659413073590, 5.891732493678457416 ) ) ;
#5682=ORIENTED_EDGE ( 'NONE', *, *, #3555, .T. ) ;
#5686=CARTESIAN_POINT ( 'NONE',  ( 26.77784341583515371, 282.2553694771634696, 10.88892170791772251 ) ) ;
#5687=VECTOR ( 'NONE', #10828, 1000.000000000000000 ) ;
#5704=EDGE_LOOP ( 'NONE', ( #8739, #11969, #10484, #13439 ) ) ;
#5708=CARTESIAN_POINT ( 'NONE',  ( 0.000000000000000000, 262.0000000000000000, -45.00000000000000711 ) ) ;
#5730=DIRECTION ( 'NONE',  ( 0.000000000000000000, 1.000000000000000000, 0.000000000000000000 ) ) ;
#5759=CARTESIAN_POINT ( 'NONE',  ( 20.00000000000000000, 312.0000000000000568, 2.500000000000002220 ) ) ;
#5770=CARTESIAN_POINT ( 'NONE',  ( 20.00000000000000000, 312.0000000000000568, -2.499999999999999556 ) ) ;
#5772=EDGE_CURVE ( 'NONE', #16375, #4102, #6205, .T. ) ;
#5793=ADVANCED_FACE ( 'NONE', ( #16003 ), #3542, .T. ) ;
#5825=ORIENTED_EDGE ( 'NONE', *, *, #11432, .T. ) ;
#5864=EDGE_CURVE ( 'NONE', #10042, #5006, #12390, .T. ) ;
#5921=VECTOR ( 'NONE', #1580, 1000.000000000000000 ) ;
#5938=DIRECTION ( 'NONE',  ( -1.000000000000000000, 0.000000000000000000, 1.734723475976807094E-17 ) ) ;
#5943=CARTESIAN_POINT ( 'NONE',  ( 0.000000000000000000, 262.0000000000000000, 0.000000000000000000 ) ) ;
#5947=CIRCLE ( 'NONE', #13099, 45.00000000000000711 ) ;
#5966=CARTESIAN_POINT ( 'NONE',  ( -21.32168401022832782, 284.4942466288908918, -8.160842005118960074 ) ) ;
#5972=SPHERICAL_SURFACE ( 'NONE', #11095, 5.000000000000000000 ) ;
#5989=EDGE_CURVE ( 'NONE', #13460, #891, #16425, .T. ) ;
#6002=CIRCLE ( 'NONE', #8107, 90.84711083310548929 ) ;
#6006=FACE_OUTER_BOUND ( 'NONE', #1748, .T. ) ;
#6038=CIRCLE ( 'NONE', #7873, 5.000000000000000888 ) ;
#6040=AXIS2_PLACEMENT_3D ( 'NONE', #3761, #8905, #3 ) ;
#6050=ADVANCED_FACE ( 'NONE', ( #3190 ), #6706, .T. ) ;
#6053=CARTESIAN_POINT ( 'NONE',  ( -25.25536947722673986, 285.3889217077648368, -3.010738954466189554 ) ) ;
#6092=( BOUNDED_SURFACE ( )  B_SPLINE_SURFACE ( 3, 2, ( 
 ( #15579, #10432, #13164 ),
 ( #15488, #13247, #8258 ),
 ( #6870, #14397, #9513 ),
 ( #2943, #593, #15659 ),
 ( #4112, #3106, #5686 ),
 ( #9182, #9347, #13323 ),
 ( #13006, #11831, #5613 ),
 ( #14246, #3019, #1774 ),
 ( #11920, #6943, #14473 ),
 ( #5453, #7932, #9426 ),
 ( #11675, #10756, #520 ),
 ( #10678, #6702, #1923 ),
 ( #4360, #15730, #8181 ),
 ( #11752, #11995, #353 ),
 ( #10517, #4205, #8010 ),
 ( #13084, #1689, #10841 ),
 ( #12244, #4529, #15981 ),
 ( #2011, #16156, #6108 ) ),
 .UNSPECIFIED., .F., .F., .F. ) 
 B_SPLINE_SURFACE_WITH_KNOTS ( ( 4, 2, 2, 2, 2, 2, 2, 2, 4 ),
 ( 3, 3 ),
 ( 4.712388980384689674, 4.908738521234051966, 5.105088062083414258, 5.301437602932775661, 5.497787143782137953, 5.694136684631500245, 5.890486225480861648, 6.086835766330223940, 6.283185307179586232 ),
 ( 0.000000000000000000, 1.000000000000000000 ),
 .UNSPECIFIED. ) 
 GEOMETRIC_REPRESENTATION_ITEM ( )  RATIONAL_B_SPLINE_SURFACE ( (
 ( 1.000000000000000000, 1.000000000000000000, 1.000000000000000000),
 ( 1.000000000000000000, 1.000000000000000000, 1.000000000000000000),
 ( 1.000000000000000000, 0.9967613244521891236, 1.000000000000000000),
 ( 1.000000000000000000, 0.9841171504955514848, 1.000000000000000000),
 ( 1.000000000000000000, 0.9747108043452729076, 1.000000000000000000),
 ( 1.000000000000000000, 0.9506740354170398755, 1.000000000000000000),
 ( 1.000000000000000000, 0.9360421842396522418, 1.000000000000000000),
 ( 1.000000000000000000, 0.9031650994467438354, 1.000000000000000000),
 ( 1.000000000000000000, 0.8849191470849314678, 1.000000000000000000),
 ( 1.000000000000000000, 0.8471316604839481679, 1.000000000000000000),
 ( 1.000000000000000000, 0.8275942695274859373, 1.000000000000000000),
 ( 1.000000000000000000, 0.7902180087158534594, 1.000000000000000000),
 ( 1.000000000000000000, 0.7723968217384532542, 1.000000000000000000),
 ( 1.000000000000000000, 0.7418334179587526833, 1.000000000000000000),
 ( 1.000000000000000000, 0.7291288939600225616, 1.000000000000000000),
 ( 1.000000000000000000, 0.7117460025832956783, 1.000000000000000000),
 ( 1.000000000000000000, 0.7070717283366861894, 1.000000000000000000),
 ( 1.000000000000000000, 0.7071067811865476838, 1.000000000000000000) ) ) 
 REPRESENTATION_ITEM ( '' )  SURFACE ( )  );
#6093=LINE ( 'NONE', #7566, #12388 ) ;
#6094=CARTESIAN_POINT ( 'NONE',  ( -20.00000000000000355, 287.0000000000000568, -7.499999999999999112 ) ) ;
#6108=CARTESIAN_POINT ( 'NONE',  ( 20.00000000000000000, 287.0000000000000568, 7.500000000000000888 ) ) ;
#6124=ADVANCED_FACE ( 'NONE', ( #15584 ), #13010, .T. ) ;
#6145=DIRECTION ( 'NONE',  ( 1.000000000000000000, -0.000000000000000000, -1.734723475976807094E-17 ) ) ;
#6161=CARTESIAN_POINT ( 'NONE',  ( 1.096031118883500133E-14, 272.0000000000000000, -89.49773270518483059 ) ) ;
#6174=ORIENTED_EDGE ( 'NONE', *, *, #14672, .F. ) ;
#6188=FACE_OUTER_BOUND ( 'NONE', #10997, .T. ) ;
#6202=CARTESIAN_POINT ( 'NONE',  ( -20.00000000000000355, 307.0000000000000568, 2.500000000000001332 ) ) ;
#6205=LINE ( 'NONE', #16334, #15534 ) ;
#6210=CARTESIAN_POINT ( 'NONE',  ( -25.00000000000000711, 286.6727470533916176, -2.499999999998864908 ) ) ;
#6211=AXIS2_PLACEMENT_3D ( 'NONE', #2237, #8484, #12304 ) ;
#6216=DIRECTION ( 'NONE',  ( -0.000000000000000000, 1.000000000000000000, 0.000000000000000000 ) ) ;
#6217=DIRECTION ( 'NONE',  ( 2.312964634635742464E-16, 0.000000000000000000, -1.000000000000000000 ) ) ;
#6228=EDGE_CURVE ( 'NONE', #9704, #16375, #13429, .T. ) ;
#6255=ORIENTED_EDGE ( 'NONE', *, *, #3159, .T. ) ;
#6274=AXIS2_PLACEMENT_3D ( 'NONE', #14262, #3203, #13024 ) ;
#6289=CARTESIAN_POINT ( 'NONE',  ( -25.00000000000000355, 287.0000000000000568, -12.49999999999999822 ) ) ;
#6296=CARTESIAN_POINT ( 'NONE',  ( -30.00000000000000711, 282.0000000000000000, -12.49999999999999822 ) ) ;
#6309=VECTOR ( 'NONE', #14001, 1000.000000000000000 ) ;
#6311=CIRCLE ( 'NONE', #1247, 5.000000000000000000 ) ;
#6313=FILL_AREA_STYLE ('',( #2466 ) ) ;
#6324=CARTESIAN_POINT ( 'NONE',  ( -20.00000000000000355, 307.0000000000000568, -7.499999999999999112 ) ) ;
#6332=FACE_OUTER_BOUND ( 'NONE', #14444, .T. ) ;
#6354=DIRECTION ( 'NONE',  ( 0.000000000000000000, 0.9848077530122080203, 0.1736481776669307198 ) ) ;
#6367=CARTESIAN_POINT ( 'NONE',  ( 25.03223043949687820, 286.3455096218830249, -2.564460878999441196 ) ) ;
#6386=CARTESIAN_POINT ( 'NONE',  ( -25.00000000000000355, 287.0000000000000568, 12.50000000000000000 ) ) ;
#6387=CARTESIAN_POINT ( 'NONE',  ( -25.00000000000000355, 312.0000000000000568, 2.500000000000001332 ) ) ;
#6447=CARTESIAN_POINT ( 'NONE',  ( 25.00000000000000711, 287.0000000000000000, -7.500000000000000888 ) ) ;
#6491=CYLINDRICAL_SURFACE ( 'NONE', #12180, 40.00000000000000000 ) ;
#6524=EDGE_CURVE ( 'NONE', #3201, #6897, #5115, .T. ) ;
#6528=CARTESIAN_POINT ( 'NONE',  ( 25.25536947722733672, 285.3889217077634726, -3.010738954466163353 ) ) ;
#6584=CARTESIAN_POINT ( 'NONE',  ( 0.000000000000000000, 267.0000000000000000, 0.000000000000000000 ) ) ;
#6649=AXIS2_PLACEMENT_3D ( 'NONE', #728, #5730, #10880 ) ;
#6676=ORIENTED_EDGE ( 'NONE', *, *, #14174, .F. ) ;
#6698=VERTEX_POINT ( 'NONE', #5759 ) ;
#6702=CARTESIAN_POINT ( 'NONE',  ( 24.78235906514067111, 286.0218276482190731, 7.282359065130366460 ) ) ;
#6703=CARTESIAN_POINT ( 'NONE',  ( -30.00000000000000711, 282.0000000000000000, 12.50000000000000000 ) ) ;
#6706=CYLINDRICAL_SURFACE ( 'NONE', #2812, 5.000000000000000000 ) ;
#6712=EDGE_CURVE ( 'NONE', #9704, #1226, #9580, .T. ) ;
#6723=ADVANCED_FACE ( 'NONE', ( #6006 ), #12046, .T. ) ;
#6765=ORIENTED_EDGE ( 'NONE', *, *, #5989, .T. ) ;
#6767=DIRECTION ( 'NONE',  ( 1.000000000000000000, -0.000000000000000000, 1.224646799147353207E-16 ) ) ;
#6783=CARTESIAN_POINT ( 'NONE',  ( 20.00000000000000000, 307.0000000000000568, 7.500000000000002665 ) ) ;
#6788=CARTESIAN_POINT ( 'NONE',  ( -24.86904120090709469, 286.8604097559688739, 7.369041200906232270 ) ) ;
#6801=CARTESIAN_POINT ( 'NONE',  ( 0.000000000000000000, 267.0000000000000000, -40.00000000000000000 ) ) ;
#6813=AXIS2_PLACEMENT_3D ( 'NONE', #15962, #827, #13790 ) ;
#6835=ADVANCED_FACE ( 'NONE', ( #8731 ), #16296, .T. ) ;
#6852=CARTESIAN_POINT ( 'NONE',  ( 19.99999999999999645, 307.0000000000000568, -2.499999999999999556 ) ) ;
#6857=DIRECTION ( 'NONE',  ( 0.000000000000000000, 0.000000000000000000, 1.000000000000000000 ) ) ;
#6870=CARTESIAN_POINT ( 'NONE',  ( 29.34550962211229930, 282.0322304394513253, 11.19101924422353811 ) ) ;
#6891=CIRCLE ( 'NONE', #233, 79.49773270518484480 ) ;
#6897=VERTEX_POINT ( 'NONE', #3914 ) ;
#6943=CARTESIAN_POINT ( 'NONE',  ( 25.48725218877856946, 284.2907069533055733, 7.987252188778913187 ) ) ;
#6944=CARTESIAN_POINT ( 'NONE',  ( -29.34549410641294287, 282.0000000000000000, 12.17274705320727257 ) ) ;
#6972=EDGE_LOOP ( 'NONE', ( #13707, #7553, #1409, #3552 ) ) ;
#6990=ORIENTED_EDGE ( 'NONE', *, *, #10730, .F. ) ;
#7009=AXIS2_PLACEMENT_3D ( 'NONE', #3245, #4671, #12227 ) ;
#7011=VERTEX_POINT ( 'NONE', #3749 ) ;
#7027=ADVANCED_FACE ( 'NONE', ( #11644 ), #10474, .F. ) ;
#7053=DIRECTION ( 'NONE',  ( 1.000000000000000000, -0.000000000000000000, 0.000000000000000000 ) ) ;
#7060=AXIS2_PLACEMENT_3D ( 'NONE', #944, #10857, #12261 ) ;
#7066=MECHANICAL_DESIGN_GEOMETRIC_PRESENTATION_REPRESENTATION('',(#3346),#5233);
#7080=CARTESIAN_POINT ( 'NONE',  ( 4.898587196589413026E-15, 262.0000000000000000, 40.00000000000000000 ) ) ;
#7089=CARTESIAN_POINT ( 'NONE',  ( 9.735664389687646693E-15, 262.0000000000000000, -79.49773270518484480 ) ) ;
#7097=CIRCLE ( 'NONE', #3108, 2.000000000000001776 ) ;
#7136=ORIENTED_EDGE ( 'NONE', *, *, #5371, .F. ) ;
#7143=DIRECTION ( 'NONE',  ( 1.000000000000000000, -0.000000000000000000, -1.734723475976807094E-17 ) ) ;
#7162=EDGE_CURVE ( 'NONE', #12621, #13460, #395, .T. ) ;
#7189=DIRECTION ( 'NONE',  ( -0.000000000000000000, -0.000000000000000000, -1.000000000000000000 ) ) ;
#7193=ORIENTED_EDGE ( 'NONE', *, *, #10477, .T. ) ;
#7207=CARTESIAN_POINT ( 'NONE',  ( -30.00000000000000711, 282.0000000000000000, -12.49999999999999822 ) ) ;
#7217=CARTESIAN_POINT ( 'NONE',  ( -25.00000000000000355, 312.0000000000000568, 7.500000000000001776 ) ) ;
#7238=VERTEX_POINT ( 'NONE', #887 ) ;
#7265=DIRECTION ( 'NONE',  ( 0.000000000000000000, 0.000000000000000000, -1.000000000000000000 ) ) ;
#7268=CARTESIAN_POINT ( 'NONE',  ( -25.00000000000000711, 286.6727470533916176, 2.499999999998866684 ) ) ;
#7295=CARTESIAN_POINT ( 'NONE',  ( -26.02446187185519832, 283.9500510409137632, -4.548923743721432267 ) ) ;
#7310=CARTESIAN_POINT ( 'NONE',  ( 0.000000000000000000, 280.0000000000000000, 88.87749532708107836 ) ) ;
#7328=DIRECTION ( 'NONE',  ( 1.000000000000000000, 0.000000000000000000, 0.000000000000000000 ) ) ;
#7329=CIRCLE ( 'NONE', #134, 5.000000000000000888 ) ;
#7353=DIRECTION ( 'NONE',  ( 0.000000000000000000, 0.000000000000000000, -1.000000000000000000 ) ) ;
#7354=CARTESIAN_POINT ( 'NONE',  ( 24.99999999999999645, 287.0000000000000568, 7.500000000000002665 ) ) ;
#7357=VECTOR ( 'NONE', #8504, 1000.000000000000000 ) ;
#7379=CARTESIAN_POINT ( 'NONE',  ( -26.40559293885987913, 283.2826504366940412, -8.905592938856969454 ) ) ;
#7384=CIRCLE ( 'NONE', #8188, 87.81953344283027718 ) ;
#7397=ORIENTED_EDGE ( 'NONE', *, *, #12457, .T. ) ;
#7400=ORIENTED_EDGE ( 'NONE', *, *, #14008, .F. ) ;
#7405=ORIENTED_EDGE ( 'NONE', *, *, #2245, .F. ) ;
#7430=ADVANCED_BREP_SHAPE_REPRESENTATION ( '', ( #3187, #15812 ), #9193 ) ;
#7431=STYLED_ITEM ( 'NONE', ( #16272 ), #3187 ) ;
#7456=CARTESIAN_POINT ( 'NONE',  ( -23.39173249367811636, 283.2330659413073590, -9.195866246827240076 ) ) ;
#7462=DIRECTION ( 'NONE',  ( 1.000000000000000000, 0.000000000000000000, 0.000000000000000000 ) ) ;
#7481=CARTESIAN_POINT ( 'NONE',  ( -20.00000000000000355, 287.0000000000000568, -2.499999999999998668 ) ) ;
#7514=EDGE_LOOP ( 'NONE', ( #7397, #11144, #13622, #15005 ) ) ;
#7516=ORIENTED_EDGE ( 'NONE', *, *, #5772, .F. ) ;
#7522=DIRECTION ( 'NONE',  ( -1.000000000000000000, 0.000000000000000000, 1.734723475976807094E-17 ) ) ;
#7532=CARTESIAN_POINT ( 'NONE',  ( -26.77784341583514305, 282.2553694771637538, -10.88892170791705105 ) ) ;
#7539=ORIENTED_EDGE ( 'NONE', *, *, #16267, .F. ) ;
#7540=LINE ( 'NONE', #15174, #2041 ) ;
#7542=CARTESIAN_POINT ( 'NONE',  ( 9.735664389687646693E-15, 272.0000000000000000, -79.49773270518484480 ) ) ;
#7553=ORIENTED_EDGE ( 'NONE', *, *, #9270, .F. ) ;
#7559=DIRECTION ( 'NONE',  ( 0.000000000000000000, 1.000000000000000000, 0.000000000000000000 ) ) ;
#7561=CARTESIAN_POINT ( 'NONE',  ( -25.00000000000000355, 287.0000000000000568, 7.500000000000001776 ) ) ;
#7564=DIRECTION ( 'NONE',  ( 0.000000000000000000, 1.000000000000000000, 0.000000000000000000 ) ) ;
#7566=CARTESIAN_POINT ( 'NONE',  ( 4.898587196589413026E-15, 267.0000000000000000, 40.00000000000000000 ) ) ;
#7606=CLOSED_SHELL ( 'NONE', ( #6835, #7633, #15971, #15864, #14832, #6124, #12084, #4618, #1329, #846, #1938, #12715, #15846, #9516, #13472, #7027, #6723, #2522, #12585, #3172, #630, #4592, #9583, #14095, #11016, #10190, #12521, #6050, #5793, #2602, #14940, #4707, #14213, #4513, #785, #13614, #13408, #15263, #15776, #7823, #2584, #10328 ) ) ;
#7624=DIRECTION ( 'NONE',  ( 0.000000000000000000, -1.000000000000000000, 0.000000000000000000 ) ) ;
#7625=DIRECTION ( 'NONE',  ( -1.000000000000000000, 0.000000000000000000, -2.312964634635741971E-16 ) ) ;
#7633=ADVANCED_FACE ( 'NONE', ( #10376 ), #15433, .F. ) ;
#7637=CARTESIAN_POINT ( 'NONE',  ( -20.00000000000000355, 307.0000000000000568, 2.500000000000001332 ) ) ;
#7639=CARTESIAN_POINT ( 'NONE',  ( -20.00000000000000355, 287.0000000000000568, 7.500000000000001776 ) ) ;
#7653=CYLINDRICAL_SURFACE ( 'NONE', #4490, 5.000000000000000000 ) ;
#7654=DIRECTION ( 'NONE',  ( 0.000000000000000000, 0.000000000000000000, -1.000000000000000000 ) ) ;
#7656=CARTESIAN_POINT ( 'NONE',  ( -20.00000000000000355, 312.0000000000000568, 7.500000000000001776 ) ) ;
#7684=VERTEX_POINT ( 'NONE', #11698 ) ;
#7688=CARTESIAN_POINT ( 'NONE',  ( 26.69586624684728093, 283.2330659412872933, -5.891732493678564886 ) ) ;
#7690=CARTESIAN_POINT ( 'NONE',  ( 0.000000000000000000, 267.0000000000000000, 0.000000000000000000 ) ) ;
#7704=CARTESIAN_POINT ( 'NONE',  ( 19.99999999999999645, 307.0000000000000568, -2.499999999999999556 ) ) ;
#7705=DIRECTION ( 'NONE',  ( 0.000000000000000000, 0.000000000000000000, 1.000000000000000000 ) ) ;
#7738=ORIENTED_EDGE ( 'NONE', *, *, #13650, .F. ) ;
#7764=CARTESIAN_POINT ( 'NONE',  ( 20.31983351293479956, 285.7035871579556670, -7.659916756470847687 ) ) ;
#7767=FACE_OUTER_BOUND ( 'NONE', #21, .T. ) ;
#7805=VECTOR ( 'NONE', #14366, 1000.000000000000000 ) ;
#7812=DIRECTION ( 'NONE',  ( 0.000000000000000000, -1.000000000000000000, 0.000000000000000000 ) ) ;
#7814=CARTESIAN_POINT ( 'NONE',  ( 0.000000000000000000, 272.0000000000000000, 79.49773270518484480 ) ) ;
#7823=ADVANCED_FACE ( 'NONE', ( #11508, #7767 ), #12837, .T. ) ;
#7845=CARTESIAN_POINT ( 'NONE',  ( 25.15991675647082815, 285.7035871579557806, -2.819833512935952413 ) ) ;
#7847=CARTESIAN_POINT ( 'NONE',  ( -25.00000000000000355, 307.0000000000000568, 7.500000000000001776 ) ) ;
#7849=CARTESIAN_POINT ( 'NONE',  ( -25.48725218878006160, 284.2907069533295612, 7.987252188781084783 ) ) ;
#7862=VECTOR ( 'NONE', #5558, 1000.000000000000000 ) ;
#7873=AXIS2_PLACEMENT_3D ( 'NONE', #9929, #7189, #14983 ) ;
#7878=ORIENTED_EDGE ( 'NONE', *, *, #14773, .F. ) ;
#7881=VERTEX_POINT ( 'NONE', #12142 ) ;
#7900=DIRECTION ( 'NONE',  ( 0.000000000000000000, 0.000000000000000000, -1.000000000000000000 ) ) ;
#7905=CARTESIAN_POINT ( 'NONE',  ( 24.99999999999999645, 307.0000000000000568, 7.500000000000002665 ) ) ;
#7929=CARTESIAN_POINT ( 'NONE',  ( 25.56848793686463139, 282.5058351977235134, -10.28424396843206523 ) ) ;
#7932=CARTESIAN_POINT ( 'NONE',  ( 25.07567824489208164, 285.0109613521088932, 7.575678244891727253 ) ) ;
#7933=CARTESIAN_POINT ( 'NONE',  ( -29.01527194596179271, 282.0655843567852799, 11.51527194596495463 ) ) ;
#7945=ORIENTED_EDGE ( 'NONE', *, *, #16408, .T. ) ;
#7948=EDGE_LOOP ( 'NONE', ( #2956, #8879 ) ) ;
#8003=VERTEX_POINT ( 'NONE', #7080 ) ;
#8010=CARTESIAN_POINT ( 'NONE',  ( 20.31983351293711237, 285.7035871579557238, 7.659916756470837917 ) ) ;
#8011=CARTESIAN_POINT ( 'NONE',  ( -20.51073895446497986, 285.3889217077648368, 7.755369477226736308 ) ) ;
#8014=CARTESIAN_POINT ( 'NONE',  ( -4.336808689942015887E-17, 307.0000000000000568, -2.499999999999999112 ) ) ;
#8024=LINE ( 'NONE', #6801, #7862 ) ;
#8040=EDGE_CURVE ( 'NONE', #11148, #8474, #15577, .T. ) ;
#8042=EDGE_LOOP ( 'NONE', ( #11410, #15131, #6990 ) ) ;
#8071=CARTESIAN_POINT ( 'NONE',  ( 30.00000000000000000, 282.0000000000000000, 12.50000000000000178 ) ) ;
#8092=CARTESIAN_POINT ( 'NONE',  ( -26.40559293885987913, 283.2826504366940981, 8.905592938858424290 ) ) ;
#8099=AXIS2_PLACEMENT_3D ( 'NONE', #11523, #6217, #7625 ) ;
#8107=AXIS2_PLACEMENT_3D ( 'NONE', #13359, #8784, #7705 ) ;
#8114=AXIS2_PLACEMENT_3D ( 'NONE', #1613, #11756, #11836 ) ;
#8137=AXIS2_PLACEMENT_3D ( 'NONE', #8748, #10008, #15065 ) ;
#8155=VECTOR ( 'NONE', #10819, 1000.000000000000000 ) ;
#8162=CARTESIAN_POINT ( 'NONE',  ( 19.99999999999999289, 287.0000000000000568, 7.500000000000002665 ) ) ;
#8181=CARTESIAN_POINT ( 'NONE',  ( 21.01167039530811209, 284.7842439685853719, 8.005835197659997959 ) ) ;
#8188=AXIS2_PLACEMENT_3D ( 'NONE', #3974, #14101, #11296 ) ;
#8209=VERTEX_POINT ( 'NONE', #2232 ) ;
#8216=VECTOR ( 'NONE', #1985, 1000.000000000000000 ) ;
#8224=CARTESIAN_POINT ( 'NONE',  ( -20.00000000000000355, 287.0000000000000568, 2.500000000000000444 ) ) ;
#8227=VERTEX_POINT ( 'NONE', #12223 ) ;
#8234=DIRECTION ( 'NONE',  ( 0.000000000000000000, 0.000000000000000000, 1.000000000000000000 ) ) ;
#8238=CARTESIAN_POINT ( 'NONE',  ( 19.99999999999999645, 307.0000000000000568, 2.500000000000002220 ) ) ;
#8255=ORIENTED_EDGE ( 'NONE', *, *, #5509, .F. ) ;
#8258=CARTESIAN_POINT ( 'NONE',  ( 29.34549410641285405, 282.0000000000000000, 12.17274705320883754 ) ) ;
#8272=VERTEX_POINT ( 'NONE', #12692 ) ;
#8316=DIRECTION ( 'NONE',  ( -1.000000000000000000, 0.000000000000000000, -2.602085213965210149E-16 ) ) ;
#8326=CIRCLE ( 'NONE', #4353, 5.000000000000000000 ) ;
#8334=CARTESIAN_POINT ( 'NONE',  ( 19.99999999999999645, 307.0000000000000568, -2.499999999999999556 ) ) ;
#8367=ORIENTED_EDGE ( 'NONE', *, *, #10730, .T. ) ;
#8381=CIRCLE ( 'NONE', #9723, 2.000000000000001776 ) ;
#8389=ORIENTED_EDGE ( 'NONE', *, *, #1857, .F. ) ;
#8403=( BOUNDED_CURVE ( )  B_SPLINE_CURVE ( 3, ( #9906, #14960, #3333, #6094 ),
 .UNSPECIFIED., .F., .F. ) 
 B_SPLINE_CURVE_WITH_KNOTS ( ( 4, 4 ),
 ( 1.570796326794897002, 3.141592653589793116 ),
 .UNSPECIFIED. ) 
 CURVE ( )  GEOMETRIC_REPRESENTATION_ITEM ( )  RATIONAL_B_SPLINE_CURVE ( ( 1.000000000000000000, 0.8047378541243650485, 0.8047378541243650485, 1.000000000000000000 ) ) 
 REPRESENTATION_ITEM ( '' )  );
#8417=EDGE_LOOP ( 'NONE', ( #16010, #5030, #2787, #15325 ) ) ;
#8474=VERTEX_POINT ( 'NONE', #14801 ) ;
#8479=ORIENTED_EDGE ( 'NONE', *, *, #10513, .F. ) ;
#8484=DIRECTION ( 'NONE',  ( 1.734723475976807094E-17, -0.000000000000000000, 1.000000000000000000 ) ) ;
#8499=( BOUNDED_CURVE ( )  B_SPLINE_CURVE ( 3, ( #12354, #11127, #16187, #12447 ),
 .UNSPECIFIED., .F., .F. ) 
 B_SPLINE_CURVE_WITH_KNOTS ( ( 4, 4 ),
 ( 0.000000000000000000, 1.570796326794896336 ),
 .UNSPECIFIED. ) 
 CURVE ( )  GEOMETRIC_REPRESENTATION_ITEM ( )  RATIONAL_B_SPLINE_CURVE ( ( 1.000000000000000000, 0.8047378541243650485, 0.8047378541243650485, 1.000000000000000000 ) ) 
 REPRESENTATION_ITEM ( '' )  );
#8504=DIRECTION ( 'NONE',  ( 2.312964634635742464E-16, 0.000000000000000000, -1.000000000000000000 ) ) ;
#8518=CARTESIAN_POINT ( 'NONE',  ( 0.000000000000000000, 267.0000000000000000, -45.00000000000000711 ) ) ;
#8524=CARTESIAN_POINT ( 'NONE',  ( -25.56848793686307175, 282.5058351977235134, -10.28424396843205457 ) ) ;
#8538=EDGE_CURVE ( 'NONE', #11555, #10428, #1154, .T. ) ;
#8556=CARTESIAN_POINT ( 'NONE',  ( 1.106078086759636654E-14, 273.6527036446661896, -89.78914894885470233 ) ) ;
#8560=DIRECTION ( 'NONE',  ( 1.000000000000000000, 0.000000000000000000, 0.000000000000000000 ) ) ;
#8574=FACE_OUTER_BOUND ( 'NONE', #11950, .T. ) ;
#8600=CARTESIAN_POINT ( 'NONE',  ( -27.78424396843074362, 282.5058351977240250, -8.068487936864610077 ) ) ;
#8605=ORIENTED_EDGE ( 'NONE', *, *, #14107, .T. ) ;
#8622=AXIS2_PLACEMENT_3D ( 'NONE', #2193, #3288, #12438 ) ;
#8642=CARTESIAN_POINT ( 'NONE',  ( 20.00000000000000000, 287.0000000000000568, -2.499999999999999556 ) ) ;
#8694=CARTESIAN_POINT ( 'NONE',  ( -20.31983351293596129, 285.7035871579731179, -7.659916756467383792 ) ) ;
#8699=AXIS2_PLACEMENT_3D ( 'NONE', #10051, #3731, #8877 ) ;
#8704=CARTESIAN_POINT ( 'NONE',  ( -20.00000000000000355, 312.0000000000000568, -7.499999999999999112 ) ) ;
#8710=SURFACE_SIDE_STYLE ('',( #13853 ) ) ;
#8719=DIRECTION ( 'NONE',  ( 0.000000000000000000, 0.000000000000000000, 1.000000000000000000 ) ) ;
#8731=FACE_OUTER_BOUND ( 'NONE', #8417, .T. ) ;
#8739=ORIENTED_EDGE ( 'NONE', *, *, #14807, .F. ) ;
#8742=DIRECTION ( 'NONE',  ( 0.000000000000000000, 0.000000000000000000, -1.000000000000000000 ) ) ;
#8748=CARTESIAN_POINT ( 'NONE',  ( 0.000000000000000000, 272.0000000000000000, 0.000000000000000000 ) ) ;
#8750=CIRCLE ( 'NONE', #4800, 5.000000000000000000 ) ;
#8765=ORIENTED_EDGE ( 'NONE', *, *, #4809, .F. ) ;
#8777=CARTESIAN_POINT ( 'NONE',  ( -29.34550962211183744, 282.0322304394514390, -11.19101924422352035 ) ) ;
#8784=DIRECTION ( 'NONE',  ( -0.000000000000000000, -1.000000000000000000, -0.000000000000000000 ) ) ;
#8798=DIRECTION ( 'NONE',  ( 0.000000000000000000, -1.000000000000000000, 0.000000000000000000 ) ) ;
#8805=SPHERICAL_SURFACE ( 'NONE', #3097, 5.000000000000000000 ) ;
#8832=DIRECTION ( 'NONE',  ( -0.000000000000000000, 0.000000000000000000, 1.000000000000000000 ) ) ;
#8872=FILL_AREA_STYLE ('',( #12458 ) ) ;
#8877=DIRECTION ( 'NONE',  ( 0.000000000000000000, -0.000000000000000000, 1.000000000000000000 ) ) ;
#8879=ORIENTED_EDGE ( 'NONE', *, *, #29, .T. ) ;
#8905=DIRECTION ( 'NONE',  ( 0.000000000000000000, 1.000000000000000000, 0.000000000000000000 ) ) ;
#8933=CARTESIAN_POINT ( 'NONE',  ( 24.99999979514750947, 287.0011897833099397, -7.499999667114691349 ) ) ;
#8956=EDGE_CURVE ( 'NONE', #13519, #7238, #9977, .T. ) ;
#8979=CARTESIAN_POINT ( 'NONE',  ( 30.00000000000000000, 282.0000000000000000, 12.50000000000000178 ) ) ;
#8988=EDGE_CURVE ( 'NONE', #11555, #13617, #13865, .T. ) ;
#9018=CARTESIAN_POINT ( 'NONE',  ( 30.00000000000001066, 282.0000000000000000, -12.50000000000000000 ) ) ;
#9042=DIRECTION ( 'NONE',  ( -1.000000000000000000, 0.000000000000000000, -1.734723475976806848E-16 ) ) ;
#9048=ORIENTED_EDGE ( 'NONE', *, *, #10371, .T. ) ;
#9064=CARTESIAN_POINT ( 'NONE',  ( 24.99999999999999645, 287.0000000000000568, 2.500000000000003109 ) ) ;
#9071=FACE_OUTER_BOUND ( 'NONE', #11891, .T. ) ;
#9096=CARTESIAN_POINT ( 'NONE',  ( 25.00000000000000355, 286.6727470533787709, -2.499999999998864020 ) ) ;
#9147=CARTESIAN_POINT ( 'NONE',  ( 25.00000000000000000, 312.0000000000000568, -2.499999999999997780 ) ) ;
#9177=ORIENTED_EDGE ( 'NONE', *, *, #8538, .F. ) ;
#9179=CARTESIAN_POINT ( 'NONE',  ( 26.78441608355291947, 282.9883952696292226, -9.284416083551356280 ) ) ;
#9182=CARTESIAN_POINT ( 'NONE',  ( 27.78424396843206878, 282.5058351977235134, 8.068487936863856902 ) ) ;
#9190=PRODUCT_DEFINITION_SHAPE ( 'NONE', 'NONE',  #4279 ) ;
#9193=( GEOMETRIC_REPRESENTATION_CONTEXT ( 3 ) GLOBAL_UNCERTAINTY_ASSIGNED_CONTEXT ( ( #265 ) ) GLOBAL_UNIT_ASSIGNED_CONTEXT ( ( #1967, #3484, #2636 ) ) REPRESENTATION_CONTEXT ( 'NONE', 'WORKASPACE' ) );
#9198=CIRCLE ( 'NONE', #12651, 40.00000000000000000 ) ;
#9199=ORIENTED_EDGE ( 'NONE', *, *, #15522, .T. ) ;
#9212=VECTOR ( 'NONE', #6354, 1000.000000000000000 ) ;
#9218=EDGE_LOOP ( 'NONE', ( #14590, #1184, #1455, #6255 ) ) ;
#9223=ORIENTED_EDGE ( 'NONE', *, *, #5772, .T. ) ;
#9224=AXIS2_PLACEMENT_3D ( 'NONE', #10421, #15475, #14225 ) ;
#9244=ORIENTED_EDGE ( 'NONE', *, *, #2520, .F. ) ;
#9270=EDGE_CURVE ( 'NONE', #13515, #6698, #9382, .T. ) ;
#9271=CARTESIAN_POINT ( 'NONE',  ( -28.38892170791837799, 282.2553694771631854, 9.277843415834363228 ) ) ;
#9303=CARTESIAN_POINT ( 'NONE',  ( -20.00000000000000355, 284.0710678118655323, 7.500000000000000000 ) ) ;
#9307=CARTESIAN_POINT ( 'NONE',  ( -25.00000000000000355, 307.0000000000000568, 2.500000000000001332 ) ) ;
#9329=CARTESIAN_POINT ( 'NONE',  ( 1.088435401685436854E-14, 280.0000000000000000, -88.87749532708107836 ) ) ;
#9347=CARTESIAN_POINT ( 'NONE',  ( 26.78441608355448977, 282.9883952696292795, 9.284416083549791310 ) ) ;
#9348=CARTESIAN_POINT ( 'NONE',  ( -25.00000020635302889, 287.0011902442391261, 7.499999664676339606 ) ) ;
#9363=PLANE ( 'NONE',  #3652 ) ;
#9374=CARTESIAN_POINT ( 'NONE',  ( 0.000000000000000000, 272.0000000000000000, 0.000000000000000000 ) ) ;
#9375=EDGE_LOOP ( 'NONE', ( #2807, #14128, #11563, #2067 ) ) ;
#9382=LINE ( 'NONE', #4238, #12886 ) ;
#9388=EDGE_CURVE ( 'NONE', #81, #8272, #14997, .T. ) ;
#9392=DIRECTION ( 'NONE',  ( 0.000000000000000000, -0.000000000000000000, -1.000000000000000000 ) ) ;
#9394=DIRECTION ( 'NONE',  ( 0.000000000000000000, 1.000000000000000000, 0.000000000000000000 ) ) ;
#9396=LINE ( 'NONE', #13456, #2988 ) ;
#9408=DIRECTION ( 'NONE',  ( -6.938893903907222461E-16, -1.000000000000000000, 0.000000000000000000 ) ) ;
#9414=DIRECTION ( 'NONE',  ( 1.000000000000000000, 0.000000000000000000, 1.734723475976807094E-17 ) ) ;
#9426=CARTESIAN_POINT ( 'NONE',  ( 22.46613188259122040, 283.6958662468466059, 8.733065941287961209 ) ) ;
#9489=CIRCLE ( 'NONE', #4993, 89.78914894885470233 ) ;
#9491=LINE ( 'NONE', #7905, #8155 ) ;
#9495=DIRECTION ( 'NONE',  ( -0.000000000000000000, -1.000000000000000000, -0.000000000000000000 ) ) ;
#9513=CARTESIAN_POINT ( 'NONE',  ( 28.69101924422353989, 282.0322304394514958, 11.84550962211153724 ) ) ;
#9515=CARTESIAN_POINT ( 'NONE',  ( -23.90010208165381655, 283.0244618719127629, 9.450051040827698756 ) ) ;
#9516=ADVANCED_FACE ( 'NONE', ( #14927 ), #9711, .F. ) ;
#9531=VECTOR ( 'NONE', #11451, 1000.000000000000000 ) ;
#9539=TOROIDAL_SURFACE ( 'NONE', #11139, 88.87749532708107836, 2.000000000000000000 ) ;
#9541=FACE_OUTER_BOUND ( 'NONE', #7514, .T. ) ;
#9562=EDGE_LOOP ( 'NONE', ( #15113, #14030, #9640 ) ) ;
#9567=EDGE_CURVE ( 'NONE', #6897, #11171, #6002, .T. ) ;
#9572=ORIENTED_EDGE ( 'NONE', *, *, #5864, .T. ) ;
#9577=DIRECTION ( 'NONE',  ( 0.000000000000000000, 0.000000000000000000, -1.000000000000000000 ) ) ;
#9580=LINE ( 'NONE', #909, #5687 ) ;
#9583=ADVANCED_FACE ( 'NONE', ( #1209 ), #4985, .T. ) ;
#9607=ORIENTED_EDGE ( 'NONE', *, *, #4378, .F. ) ;
#9621=ORIENTED_EDGE ( 'NONE', *, *, #1214, .F. ) ;
#9625=CARTESIAN_POINT ( 'NONE',  ( -2.168404344971008868E-16, 282.0000000000000000, -12.50000000000000000 ) ) ;
#9640=ORIENTED_EDGE ( 'NONE', *, *, #5400, .F. ) ;
#9669=DIRECTION ( 'NONE',  ( 0.000000000000000000, -1.000000000000000000, 0.000000000000000000 ) ) ;
#9677=EDGE_CURVE ( 'NONE', #13617, #3799, #3963, .T. ) ;
#9683=AXIS2_PLACEMENT_3D ( 'NONE', #12863, #10298, #11530 ) ;
#9704=VERTEX_POINT ( 'NONE', #4898 ) ;
#9711=PLANE ( 'NONE',  #656 ) ;
#9717=DIRECTION ( 'NONE',  ( -1.000000000000000000, 0.000000000000000000, 0.000000000000000000 ) ) ;
#9723=AXIS2_PLACEMENT_3D ( 'NONE', #9329, #6767, #14380 ) ;
#9729=CARTESIAN_POINT ( 'NONE',  ( 0.000000000000000000, 262.0000000000000000, 0.000000000000000000 ) ) ;
#9731=ORIENTED_EDGE ( 'NONE', *, *, #15309, .T. ) ;
#9735=AXIS2_PLACEMENT_3D ( 'NONE', #4341, #4182, #10734 ) ;
#9745=CARTESIAN_POINT ( 'NONE',  ( 0.000000000000000000, 280.0000000000000000, 0.000000000000000000 ) ) ;
#9790=CARTESIAN_POINT ( 'NONE',  ( -25.66084200511936686, 284.4942466288902096, -3.821684010227674566 ) ) ;
#9803=CARTESIAN_POINT ( 'NONE',  ( -25.00000000000000355, 307.0000000000000568, 7.500000000000001776 ) ) ;
#9838=VERTEX_POINT ( 'NONE', #368 ) ;
#9855=EDGE_LOOP ( 'NONE', ( #8255, #14530, #13181 ) ) ;
#9860=DIRECTION ( 'NONE',  ( 0.000000000000000000, 1.000000000000000000, 0.000000000000000000 ) ) ;
#9866=CARTESIAN_POINT ( 'NONE',  ( -28.07127062163582920, 282.3184422169439927, -10.57127062163423403 ) ) ;
#9906=CARTESIAN_POINT ( 'NONE',  ( -30.00000000000000711, 282.0000000000000000, -12.49999999999999822 ) ) ;
#9929=CARTESIAN_POINT ( 'NONE',  ( -20.00000000000000355, 307.0000000000000568, 2.500000000000001332 ) ) ;
#9947=CARTESIAN_POINT ( 'NONE',  ( -20.51073895446497986, 285.3889217077648368, -7.755369477226732755 ) ) ;
#9950=EDGE_LOOP ( 'NONE', ( #15378, #11558 ) ) ;
#9977=LINE ( 'NONE', #3906, #5463 ) ;
#9984=DIRECTION ( 'NONE',  ( 0.000000000000000000, 0.000000000000000000, -1.000000000000000000 ) ) ;
#10008=DIRECTION ( 'NONE',  ( 0.000000000000000000, 1.000000000000000000, 0.000000000000000000 ) ) ;
#10031=FACE_BOUND ( 'NONE', #9950, .T. ) ;
#10038=CARTESIAN_POINT ( 'NONE',  ( -28.69101924422432148, 282.0322304394514390, -11.84550962211183389 ) ) ;
#10042=VERTEX_POINT ( 'NONE', #5708 ) ;
#10048=DIRECTION ( 'NONE',  ( 0.000000000000000000, -1.000000000000000000, 0.000000000000000000 ) ) ;
#10051=CARTESIAN_POINT ( 'NONE',  ( 0.000000000000000000, 272.0000000000000000, 0.000000000000000000 ) ) ;
#10062=ORIENTED_EDGE ( 'NONE', *, *, #1214, .T. ) ;
#10077=EDGE_CURVE ( 'NONE', #1042, #12043, #1473, .T. ) ;
#10079=COLOUR_RGB ( '', 0.66274510, 0.83137255, 0.94901961) ;
#10105=CARTESIAN_POINT ( 'NONE',  ( 20.00000000000000355, 287.0000000000000568, -7.500000000000000888 ) ) ;
#10123=DIRECTION ( 'NONE',  ( 0.000000000000000000, 0.000000000000000000, -1.000000000000000000 ) ) ;
#10154=ORIENTED_EDGE ( 'NONE', *, *, #2371, .F. ) ;
#10159=DIRECTION ( 'NONE',  ( -1.000000000000000000, 0.000000000000000000, 0.000000000000000000 ) ) ;
#10184=CARTESIAN_POINT ( 'NONE',  ( 25.00000000000000355, 287.0000000000000568, -2.499999999999999556 ) ) ;
#10188=CIRCLE ( 'NONE', #3011, 5.000000000000000000 ) ;
#10190=ADVANCED_FACE ( 'NONE', ( #8574 ), #2256, .T. ) ;
#10227=CARTESIAN_POINT ( 'NONE',  ( 19.99999999999999645, 307.0000000000000568, 2.500000000000002220 ) ) ;
#10241=ORIENTED_EDGE ( 'NONE', *, *, #12818, .F. ) ;
#10258=AXIS2_PLACEMENT_3D ( 'NONE', #10583, #653, #11732 ) ;
#10265=ORIENTED_EDGE ( 'NONE', *, *, #6228, .T. ) ;
#10266=CARTESIAN_POINT ( 'NONE',  ( 27.78424396843207234, 282.5058351977235134, -8.068487936863856902 ) ) ;
#10298=DIRECTION ( 'NONE',  ( -0.000000000000000000, -1.000000000000000000, -0.000000000000000000 ) ) ;
#10306=ORIENTED_EDGE ( 'NONE', *, *, #832, .F. ) ;
#10328=ADVANCED_FACE ( 'NONE', ( #2751 ), #2925, .F. ) ;
#10337=CARTESIAN_POINT ( 'NONE',  ( -30.00000000000000711, 287.0000000000000568, 7.500000000000001776 ) ) ;
#10345=CARTESIAN_POINT ( 'NONE',  ( 25.07567824489208519, 285.0109613521088932, -7.575678244889592072 ) ) ;
#10371=EDGE_CURVE ( 'NONE', #11171, #9838, #8381, .T. ) ;
#10372=DIRECTION ( 'NONE',  ( 0.000000000000000000, 0.000000000000000000, 1.000000000000000000 ) ) ;
#10376=FACE_OUTER_BOUND ( 'NONE', #5704, .T. ) ;
#10402=ORIENTED_EDGE ( 'NONE', *, *, #10419, .F. ) ;
#10419=EDGE_CURVE ( 'NONE', #11171, #6897, #3066, .T. ) ;
#10421=CARTESIAN_POINT ( 'NONE',  ( 0.000000000000000000, 282.0000000000000000, 0.000000000000000000 ) ) ;
#10425=CARTESIAN_POINT ( 'NONE',  ( -20.00000000000000711, 287.0000000000000568, -7.500000000000000888 ) ) ;
#10426=ORIENTED_EDGE ( 'NONE', *, *, #1722, .T. ) ;
#10428=VERTEX_POINT ( 'NONE', #14541 ) ;
#10429=CARTESIAN_POINT ( 'NONE',  ( 27.49424662897629901, 282.6608420050619088, -7.488493257954151439 ) ) ;
#10432=CARTESIAN_POINT ( 'NONE',  ( 30.00000000000000000, 282.0000000000000000, 12.50000000000000178 ) ) ;
#10438=AXIS2_PLACEMENT_3D ( 'NONE', #14185, #223, #15265 ) ;
#10474=PLANE ( 'NONE',  #13637 ) ;
#10477=EDGE_CURVE ( 'NONE', #6698, #7881, #7329, .T. ) ;
#10484=ORIENTED_EDGE ( 'NONE', *, *, #15323, .T. ) ;
#10503=( BOUNDED_SURFACE ( )  B_SPLINE_SURFACE ( 3, 2, ( 
 ( #6703, #13007, #443 ),
 ( #6944, #13248, #274 ),
 ( #1776, #7933, #521 ),
 ( #3021, #4114, #15662 ),
 ( #1610, #594, #9271 ),
 ( #11753, #15731, #11921 ),
 ( #12929, #8092, #354 ),
 ( #9515, #15581, #11676 ),
 ( #2776, #7849, #5616 ),
 ( #5454, #10519, #1532 ),
 ( #10757, #15817, #5378 ),
 ( #13166, #4362, #4451 ),
 ( #14474, #14327, #2944 ),
 ( #8011, #13085, #10605 ),
 ( #1691, #6788, #11832 ),
 ( #3109, #5544, #4284 ),
 ( #14398, #9348, #7268 ),
 ( #10842, #2012, #3268 ) ),
 .UNSPECIFIED., .F., .F., .T. ) 
 B_SPLINE_SURFACE_WITH_KNOTS ( ( 4, 2, 2, 2, 2, 2, 2, 2, 4 ),
 ( 3, 3 ),
 ( 1.570796326794896558, 1.767145867644258628, 1.963495408493620697, 2.159844949342982545, 2.356194490192344837, 2.552544031041707129, 2.748893571891068976, 2.945243112740430824, 3.141592653589793116 ),
 ( 0.000000000000000000, 1.000000000000000000 ),
 .UNSPECIFIED. ) 
 GEOMETRIC_REPRESENTATION_ITEM ( )  RATIONAL_B_SPLINE_SURFACE ( (
 ( 1.000000000000000000, 1.000000000000000000, 1.000000000000000000),
 ( 1.000000000000000000, 1.000000000000000000, 1.000000000000000000),
 ( 1.000000000000000000, 0.9967613244521498217, 1.000000000000000000),
 ( 1.000000000000000000, 0.9841171504955907867, 1.000000000000000000),
 ( 1.000000000000000000, 0.9747108043452232806, 1.000000000000000000),
 ( 1.000000000000000000, 0.9506740354170890583, 1.000000000000000000),
 ( 1.000000000000000000, 0.9360421842396996484, 1.000000000000000000),
 ( 1.000000000000000000, 0.9031650994466967619, 1.000000000000000000),
 ( 1.000000000000000000, 0.8849191470854951280, 1.000000000000000000),
 ( 1.000000000000000000, 0.8471316604833825092, 1.000000000000000000),
 ( 1.000000000000000000, 0.8275942695279743244, 1.000000000000000000),
 ( 1.000000000000000000, 0.7902180087153679588, 1.000000000000000000),
 ( 1.000000000000000000, 0.7723968217385259738, 1.000000000000000000),
 ( 1.000000000000000000, 0.7418334179586800747, 1.000000000000000000),
 ( 1.000000000000000000, 0.7291288939600593100, 1.000000000000000000),
 ( 1.000000000000000000, 0.7117460025832584858, 1.000000000000000000),
 ( 1.000000000000000000, 0.7070717283367141670, 1.000000000000000000),
 ( 1.000000000000000000, 0.7071067811865475727, 1.000000000000000000) ) ) 
 REPRESENTATION_ITEM ( '' )  SURFACE ( )  );
#10513=EDGE_CURVE ( 'NONE', #15703, #11171, #1070, .T. ) ;
#10517=CARTESIAN_POINT ( 'NONE',  ( 25.15991675647091697, 285.7035871579553259, 2.819833512935955966 ) ) ;
#10519=CARTESIAN_POINT ( 'NONE',  ( -25.07567824489023778, 285.0109613520845073, 7.575678244889168411 ) ) ;
#10529=COLOUR_RGB ( '', 0.66274510, 0.83137255, 0.94901961) ;
#10556=CARTESIAN_POINT ( 'NONE',  ( -20.00000000000000355, 287.0000000000000568, 7.500000000000001776 ) ) ;
#10561=AXIS2_PLACEMENT_3D ( 'NONE', #6386, #11522, #10123 ) ;
#10572=CARTESIAN_POINT ( 'NONE',  ( -20.00000000000000355, 312.0000000000000568, 2.500000000000001332 ) ) ;
#10583=CARTESIAN_POINT ( 'NONE',  ( 0.000000000000000000, 262.0000000000000000, 0.000000000000000000 ) ) ;
#10605=CARTESIAN_POINT ( 'NONE',  ( -25.25536947722673986, 285.3889217077648368, 3.010738954466191331 ) ) ;
#10647=CARTESIAN_POINT ( 'NONE',  ( 0.000000000000000000, 272.0000000000000000, 0.000000000000000000 ) ) ;
#10663=LINE ( 'NONE', #15471, #3624 ) ;
#10678=CARTESIAN_POINT ( 'NONE',  ( 25.66084200510923807, 284.4942466289053868, 3.821684010227777595 ) ) ;
#10689=VERTEX_POINT ( 'NONE', #14873 ) ;
#10691=EDGE_LOOP ( 'NONE', ( #8479, #3735, #302, #4625 ) ) ;
#10730=EDGE_CURVE ( 'NONE', #2646, #7238, #14219, .T. ) ;
#10734=DIRECTION ( 'NONE',  ( 0.000000000000000000, 0.000000000000000000, -1.000000000000000000 ) ) ;
#10756=CARTESIAN_POINT ( 'NONE',  ( 24.93825083352558636, 285.3724546740382948, 7.438250833535430928 ) ) ;
#10757=CARTESIAN_POINT ( 'NONE',  ( -22.04892374372078834, 283.9500510409134790, 8.524461871855393724 ) ) ;
#10800=DIRECTION ( 'NONE',  ( 0.000000000000000000, 0.000000000000000000, 1.000000000000000000 ) ) ;
#10817=CIRCLE ( 'NONE', #451, 40.00000000000000000 ) ;
#10819=DIRECTION ( 'NONE',  ( -2.312964634635742464E-16, -0.000000000000000000, 1.000000000000000000 ) ) ;
#10828=DIRECTION ( 'NONE',  ( 0.000000000000000000, 1.000000000000000000, 0.000000000000000000 ) ) ;
#10834=EDGE_LOOP ( 'NONE', ( #10241, #16364, #862 ) ) ;
#10835=CARTESIAN_POINT ( 'NONE',  ( -25.00000000000000355, 287.0000000000000568, -2.499999999999998668 ) ) ;
#10841=CARTESIAN_POINT ( 'NONE',  ( 20.06446087899828967, 286.3455096218830818, 7.532230439496864882 ) ) ;
#10842=CARTESIAN_POINT ( 'NONE',  ( -20.00000000000000711, 287.0000000000000568, 7.500000000000002665 ) ) ;
#10857=DIRECTION ( 'NONE',  ( 0.000000000000000000, 1.000000000000000000, 0.000000000000000000 ) ) ;
#10880=DIRECTION ( 'NONE',  ( 0.000000000000000000, 0.000000000000000000, 1.000000000000000000 ) ) ;
#10881=CARTESIAN_POINT ( 'NONE',  ( 0.000000000000000000, 282.0000000000000000, 88.87749532708107836 ) ) ;
#10895=ORIENTED_EDGE ( 'NONE', *, *, #12457, .F. ) ;
#10967=ORIENTED_EDGE ( 'NONE', *, *, #5400, .T. ) ;
#10995=EDGE_CURVE ( 'NONE', #13460, #13519, #8499, .T. ) ;
#10997=EDGE_LOOP ( 'NONE', ( #15188, #3411, #7878, #55 ) ) ;
#11003=CARTESIAN_POINT ( 'NONE',  ( 0.000000000000000000, 267.0000000000000000, -40.00000000000000000 ) ) ;
#11015=ORIENTED_EDGE ( 'NONE', *, *, #5989, .F. ) ;
#11016=ADVANCED_FACE ( 'NONE', ( #1039 ), #14848, .T. ) ;
#11029=CARTESIAN_POINT ( 'NONE',  ( -29.67274705320269135, 282.0000000000000000, -11.84549410641580636 ) ) ;
#11038=DIRECTION ( 'NONE',  ( 0.000000000000000000, 0.000000000000000000, -1.000000000000000000 ) ) ;
#11073=DIRECTION ( 'NONE',  ( 0.000000000000000000, 0.000000000000000000, 1.000000000000000000 ) ) ;
#11080=AXIS2_PLACEMENT_3D ( 'NONE', #8642, #16295, #1073 ) ;
#11082=CIRCLE ( 'NONE', #6040, 88.87749532708107836 ) ;
#11094=CARTESIAN_POINT ( 'NONE',  ( -4.336808689942015887E-17, 312.0000000000000568, -2.499999999999999112 ) ) ;
#11095=AXIS2_PLACEMENT_3D ( 'NONE', #7704, #2296, #7462 ) ;
#11103=AXIS2_PLACEMENT_3D ( 'NONE', #5943, #4611, #12501 ) ;
#11113=VERTEX_POINT ( 'NONE', #5770 ) ;
#11116=AXIS2_PLACEMENT_3D ( 'NONE', #7637, #12703, #1303 ) ;
#11123=CARTESIAN_POINT ( 'NONE',  ( -24.78235906513968345, 286.0218276481963358, -7.282359065137699261 ) ) ;
#11127=CARTESIAN_POINT ( 'NONE',  ( 20.00000000000000711, 284.0710678118654755, -7.499999999999999112 ) ) ;
#11139=AXIS2_PLACEMENT_3D ( 'NONE', #9745, #750, #14702 ) ;
#11144=ORIENTED_EDGE ( 'NONE', *, *, #10513, .T. ) ;
#11148=VERTEX_POINT ( 'NONE', #6783 ) ;
#11158=CYLINDRICAL_SURFACE ( 'NONE', #7009, 45.00000000000000711 ) ;
#11171=VERTEX_POINT ( 'NONE', #14395 ) ;
#11172=CARTESIAN_POINT ( 'NONE',  ( -27.07106781186548261, 282.0000000000000000, -6.642135623730948346 ) ) ;
#11180=LINE ( 'NONE', #7354, #7357 ) ;
#11204=CARTESIAN_POINT ( 'NONE',  ( -22.46613188259093974, 283.6958662468272792, -8.733065941307291524 ) ) ;
#11211=DIRECTION ( 'NONE',  ( 0.000000000000000000, 0.000000000000000000, 1.000000000000000000 ) ) ;
#11220=EDGE_LOOP ( 'NONE', ( #5825, #14069 ) ) ;
#11223=ORIENTED_EDGE ( 'NONE', *, *, #2024, .T. ) ;
#11234=DIRECTION ( 'NONE',  ( 2.126576849575776229E-17, 0.9848077530122080203, -0.1736481776669307198 ) ) ;
#11248=CIRCLE ( 'NONE', #13353, 45.00000000000000711 ) ;
#11281=CARTESIAN_POINT ( 'NONE',  ( -25.00000020635302889, 287.0011902442391261, -7.499999664676337829 ) ) ;
#11285=ORIENTED_EDGE ( 'NONE', *, *, #8956, .F. ) ;
#11294=SHAPE_REPRESENTATION_RELATIONSHIP ( 'NONE' , 'NONE' ,  #329, #7430 ) ;
#11296=DIRECTION ( 'NONE',  ( 0.000000000000000000, 0.000000000000000000, 1.000000000000000000 ) ) ;
#11299=AXIS2_PLACEMENT_3D ( 'NONE', #721, #14675, #10800 ) ;
#11322=CARTESIAN_POINT ( 'NONE',  ( 0.000000000000000000, 267.0000000000000000, -45.00000000000000711 ) ) ;
#11332=CARTESIAN_POINT ( 'NONE',  ( 4.898587196589413026E-15, 267.0000000000000000, 40.00000000000000000 ) ) ;
#11354=CARTESIAN_POINT ( 'NONE',  ( 24.96465690379595515, 286.9981936728412393, -7.464656903795367171 ) ) ;
#11365=CARTESIAN_POINT ( 'NONE',  ( -26.78441608355137049, 282.9883952696293932, -9.284416083551363386 ) ) ;
#11387=EDGE_CURVE ( 'NONE', #4712, #11650, #11864, .T. ) ;
#11410=ORIENTED_EDGE ( 'NONE', *, *, #832, .T. ) ;
#11427=ORIENTED_EDGE ( 'NONE', *, *, #13650, .T. ) ;
#11432=EDGE_CURVE ( 'NONE', #13826, #9838, #11082, .T. ) ;
#11433=CARTESIAN_POINT ( 'NONE',  ( 24.76951992798385760, 286.3033656649012642, -7.269519927984439356 ) ) ;
#11437=DIRECTION ( 'NONE',  ( 0.000000000000000000, 1.000000000000000000, 0.000000000000000000 ) ) ;
#11444=CARTESIAN_POINT ( 'NONE',  ( -25.00000000000001066, 287.0000000000000000, -7.500000000000000888 ) ) ;
#11451=DIRECTION ( 'NONE',  ( -0.000000000000000000, 1.000000000000000000, -0.000000000000000000 ) ) ;
#11466=DIRECTION ( 'NONE',  ( 0.000000000000000000, 0.000000000000000000, -1.000000000000000000 ) ) ;
#11468=CARTESIAN_POINT ( 'NONE',  ( 24.99999999999999645, 287.0000000000000568, 2.500000000000003109 ) ) ;
#11469=DIRECTION ( 'NONE',  ( 0.000000000000000000, 0.000000000000000000, 1.000000000000000000 ) ) ;
#11506=CARTESIAN_POINT ( 'NONE',  ( 29.34550962211230640, 282.0322304394513253, -11.19101924422353811 ) ) ;
#11508=FACE_BOUND ( 'NONE', #714, .T. ) ;
#11511=CARTESIAN_POINT ( 'NONE',  ( -30.00000000000000711, 282.0000000000000000, 12.50000000000000000 ) ) ;
#11522=DIRECTION ( 'NONE',  ( 1.000000000000000000, -0.000000000000000000, 1.734723475976807094E-17 ) ) ;
#11523=CARTESIAN_POINT ( 'NONE',  ( 19.99999999999999645, 307.0000000000000568, 4.625929269271484533E-15 ) ) ;
#11530=DIRECTION ( 'NONE',  ( 0.000000000000000000, 0.000000000000000000, -1.000000000000000000 ) ) ;
#11533=ORIENTED_EDGE ( 'NONE', *, *, #11691, .T. ) ;
#11547=DIRECTION ( 'NONE',  ( 0.000000000000000000, -1.000000000000000000, 0.000000000000000000 ) ) ;
#11555=VERTEX_POINT ( 'NONE', #5275 ) ;
#11558=ORIENTED_EDGE ( 'NONE', *, *, #15323, .F. ) ;
#11563=ORIENTED_EDGE ( 'NONE', *, *, #3555, .F. ) ;
#11579=CIRCLE ( 'NONE', #6274, 89.78914894885470233 ) ;
#11584=ORIENTED_EDGE ( 'NONE', *, *, #199, .T. ) ;
#11591=CARTESIAN_POINT ( 'NONE',  ( 22.04892374372133546, 283.9500510408986429, -8.524461871865314677 ) ) ;
#11627=ORIENTED_EDGE ( 'NONE', *, *, #1857, .T. ) ;
#11639=CARTESIAN_POINT ( 'NONE',  ( -25.00000000000000355, 287.0000000000000568, 2.500000000000001332 ) ) ;
#11644=FACE_OUTER_BOUND ( 'NONE', #2105, .T. ) ;
#11650=VERTEX_POINT ( 'NONE', #11332 ) ;
#11664=FACE_OUTER_BOUND ( 'NONE', #11220, .T. ) ;
#11671=CARTESIAN_POINT ( 'NONE',  ( 30.00000000000000711, 282.0000000000000000, -12.50000000000000178 ) ) ;
#11673=AXIS2_PLACEMENT_3D ( 'NONE', #12534, #5075, #9042 ) ;
#11675=CARTESIAN_POINT ( 'NONE',  ( 26.02446187186531645, 283.9500510408985861, 4.548923743721332791 ) ) ;
#11676=CARTESIAN_POINT ( 'NONE',  ( -26.95005104082770231, 283.0244618719127629, 6.400102081653812114 ) ) ;
#11691=EDGE_CURVE ( 'NONE', #8272, #3201, #7097, .T. ) ;
#11697=EDGE_CURVE ( 'NONE', #13297, #7881, #9491, .T. ) ;
#11698=CARTESIAN_POINT ( 'NONE',  ( 0.000000000000000000, 262.0000000000000000, -40.00000000000000000 ) ) ;
#11732=DIRECTION ( 'NONE',  ( 0.000000000000000000, -0.000000000000000000, 1.000000000000000000 ) ) ;
#11742=CARTESIAN_POINT ( 'NONE',  ( 19.99999999999999289, 312.0000000000000568, 7.500000000000002665 ) ) ;
#11745=AXIS2_PLACEMENT_3D ( 'NONE', #9374, #14586, #621 ) ;
#11752=CARTESIAN_POINT ( 'NONE',  ( 25.25536947722714842, 285.3889217077638705, 3.010738954466165129 ) ) ;
#11753=CARTESIAN_POINT ( 'NONE',  ( -25.56848793686307175, 282.5058351977235134, 10.28424396843205635 ) ) ;
#11756=DIRECTION ( 'NONE',  ( 0.000000000000000000, 1.000000000000000000, 0.000000000000000000 ) ) ;
#11823=LINE ( 'NONE', #11742, #3800 ) ;
#11831=CARTESIAN_POINT ( 'NONE',  ( 26.40559293885843317, 283.2826504366940412, 8.905592938859888008 ) ) ;
#11832=CARTESIAN_POINT ( 'NONE',  ( -25.15991675646742465, 285.7035871579729474, 2.819833512935955078 ) ) ;
#11836=DIRECTION ( 'NONE',  ( 0.000000000000000000, 0.000000000000000000, 1.000000000000000000 ) ) ;
#11864=CIRCLE ( 'NONE', #168, 40.00000000000000000 ) ;
#11891=EDGE_LOOP ( 'NONE', ( #8389, #12010, #10426, #9621 ) ) ;
#11913=CIRCLE ( 'NONE', #14021, 5.000000000000000000 ) ;
#11920=CARTESIAN_POINT ( 'NONE',  ( 26.69586624684658105, 283.2330659412879186, 5.891732493678568439 ) ) ;
#11921=CARTESIAN_POINT ( 'NONE',  ( -27.78424396843074362, 282.5058351977240250, 8.068487936863837362 ) ) ;
#11950=EDGE_LOOP ( 'NONE', ( #4710, #6676, #10967, #349 ) ) ;
#11969=ORIENTED_EDGE ( 'NONE', *, *, #14224, .T. ) ;
#11978=CARTESIAN_POINT ( 'NONE',  ( 24.14213562373094746, 282.0000000000000000, 9.571067811865477282 ) ) ;
#11984=FACE_OUTER_BOUND ( 'NONE', #6972, .T. ) ;
#11995=CARTESIAN_POINT ( 'NONE',  ( 24.81239020281730490, 286.7275190727439167, 7.312390202817921292 ) ) ;
#12010=ORIENTED_EDGE ( 'NONE', *, *, #9677, .F. ) ;
#12043=VERTEX_POINT ( 'NONE', #6324 ) ;
#12046=TOROIDAL_SURFACE ( 'NONE', #4903, 87.81953344283027718, 2.000000000000000000 ) ;
#12053=DIRECTION ( 'NONE',  ( 0.000000000000000000, 0.000000000000000000, 1.000000000000000000 ) ) ;
#12059=DIRECTION ( 'NONE',  ( 0.000000000000000000, 1.000000000000000000, 0.000000000000000000 ) ) ;
#12076=DIRECTION ( 'NONE',  ( -1.000000000000000000, 0.000000000000000000, 1.734723475976807094E-17 ) ) ;
#12084=ADVANCED_FACE ( 'NONE', ( #3663 ), #2479, .T. ) ;
#12089=EDGE_LOOP ( 'NONE', ( #7516, #15458, #16105, #14969 ) ) ;
#12105=CIRCLE ( 'NONE', #13966, 40.00000000000000000 ) ;
#12142=CARTESIAN_POINT ( 'NONE',  ( 24.99999999999999645, 307.0000000000000568, 2.500000000000003109 ) ) ;
#12144=CARTESIAN_POINT ( 'NONE',  ( 30.00000000000000355, 282.0000000000000000, -12.50000000000000000 ) ) ;
#12146=PLANE ( 'NONE',  #6211 ) ;
#12180=AXIS2_PLACEMENT_3D ( 'NONE', #6584, #4930, #13793 ) ;
#12188=( BOUNDED_CURVE ( )  B_SPLINE_CURVE ( 3, ( #12819, #1171, #88, #1340 ),
 .UNSPECIFIED., .F., .T. ) 
 B_SPLINE_CURVE_WITH_KNOTS ( ( 4, 4 ),
 ( 4.712388980384689674, 6.283185307179586232 ),
 .UNSPECIFIED. ) 
 CURVE ( )  GEOMETRIC_REPRESENTATION_ITEM ( )  RATIONAL_B_SPLINE_CURVE ( ( 1.000000000000000000, 0.8047378541243649375, 0.8047378541243649375, 1.000000000000000000 ) ) 
 REPRESENTATION_ITEM ( '' )  );
#12189=MECHANICAL_DESIGN_GEOMETRIC_PRESENTATION_REPRESENTATION('',(#7431),#2635);
#12222=ORIENTED_EDGE ( 'NONE', *, *, #3107, .F. ) ;
#12223=CARTESIAN_POINT ( 'NONE',  ( -20.00000000000000355, 312.0000000000000568, -2.499999999999998668 ) ) ;
#12227=DIRECTION ( 'NONE',  ( 0.000000000000000000, 0.000000000000000000, -1.000000000000000000 ) ) ;
#12244=CARTESIAN_POINT ( 'NONE',  ( 25.00000000000000000, 286.6727470533782594, 2.499999999998866240 ) ) ;
#12261=DIRECTION ( 'NONE',  ( 0.000000000000000000, 0.000000000000000000, 1.000000000000000000 ) ) ;
#12268=CARTESIAN_POINT ( 'NONE',  ( -25.48725218878007936, 284.2907069533513322, -7.987252188781434725 ) ) ;
#12292=ORIENTED_EDGE ( 'NONE', *, *, #16095, .F. ) ;
#12304=DIRECTION ( 'NONE',  ( 1.000000000000000000, 0.000000000000000000, -1.734723475976807094E-17 ) ) ;
#12324=AXIS2_PLACEMENT_3D ( 'NONE', #7690, #5057, #15081 ) ;
#12351=CARTESIAN_POINT ( 'NONE',  ( -24.76951992798375102, 286.3033656649002410, -7.269519927983449037 ) ) ;
#12354=CARTESIAN_POINT ( 'NONE',  ( 19.99999999999999289, 287.0000000000000568, -7.500000000000000000 ) ) ;
#12357=AXIS2_PLACEMENT_3D ( 'NONE', #15886, #9495, #12053 ) ;
#12368=LINE ( 'NONE', #9803, #2905 ) ;
#12384=ORIENTED_EDGE ( 'NONE', *, *, #512, .T. ) ;
#12388=VECTOR ( 'NONE', #5393, 1000.000000000000000 ) ;
#12390=CIRCLE ( 'NONE', #14505, 45.00000000000000711 ) ;
#12438=DIRECTION ( 'NONE',  ( 1.000000000000000000, 0.000000000000000000, 0.000000000000000000 ) ) ;
#12445=CARTESIAN_POINT ( 'NONE',  ( -24.98849325795416121, 282.6608420050619088, -9.994246628976297231 ) ) ;
#12447=CARTESIAN_POINT ( 'NONE',  ( 30.00000000000000355, 282.0000000000000000, -12.50000000000000000 ) ) ;
#12451=FACE_OUTER_BOUND ( 'NONE', #12872, .T. ) ;
#12457=EDGE_CURVE ( 'NONE', #3201, #15703, #9489, .T. ) ;
#12458=FILL_AREA_STYLE_COLOUR ( '', #10079 ) ;
#12481=DIRECTION ( 'NONE',  ( 1.000000000000000000, 0.000000000000000000, 0.000000000000000000 ) ) ;
#12501=DIRECTION ( 'NONE',  ( 0.000000000000000000, 0.000000000000000000, 1.000000000000000000 ) ) ;
#12509=ORIENTED_EDGE ( 'NONE', *, *, #12595, .F. ) ;
#12521=ADVANCED_FACE ( 'NONE', ( #3218 ), #5972, .T. ) ;
#12523=CARTESIAN_POINT ( 'NONE',  ( -23.90010208165381655, 283.0244618719127629, -9.450051040827696980 ) ) ;
#12528=CARTESIAN_POINT ( 'NONE',  ( 19.99999999999999289, 287.0000000000000568, 7.500000000000002665 ) ) ;
#12534=CARTESIAN_POINT ( 'NONE',  ( 30.00000000000000000, 287.0000000000000568, 7.500000000000003553 ) ) ;
#12585=ADVANCED_FACE ( 'NONE', ( #12451 ), #15010, .F. ) ;
#12589=VERTEX_POINT ( 'NONE', #12528 ) ;
#12594=FACE_OUTER_BOUND ( 'NONE', #381, .T. ) ;
#12595=EDGE_CURVE ( 'NONE', #8227, #13515, #7540, .T. ) ;
#12603=CARTESIAN_POINT ( 'NONE',  ( -25.50583519766042429, 284.7842439685843487, -3.511670395308089443 ) ) ;
#12618=EDGE_CURVE ( 'NONE', #13297, #12621, #6311, .T. ) ;
#12621=VERTEX_POINT ( 'NONE', #1122 ) ;
#12625=ORIENTED_EDGE ( 'NONE', *, *, #1933, .F. ) ;
#12628=EDGE_LOOP ( 'NONE', ( #14779, #16190, #14235, #7193 ) ) ;
#12631=DIRECTION ( 'NONE',  ( -0.000000000000000000, 0.000000000000000000, 1.000000000000000000 ) ) ;
#12651=AXIS2_PLACEMENT_3D ( 'NONE', #9729, #8798, #4755 ) ;
#12679=ORIENTED_EDGE ( 'NONE', *, *, #14672, .T. ) ;
#12680=CARTESIAN_POINT ( 'NONE',  ( 29.50911996093742928, 282.0000000000000000, -12.00911996093662104 ) ) ;
#12692=CARTESIAN_POINT ( 'NONE',  ( 0.000000000000000000, 272.0000000000000000, 87.81953344283027718 ) ) ;
#12693=ORIENTED_EDGE ( 'NONE', *, *, #3159, .F. ) ;
#12700=CARTESIAN_POINT ( 'NONE',  ( 24.99999999999999645, 312.0000000000000568, 2.500000000000003109 ) ) ;
#12703=DIRECTION ( 'NONE',  ( 0.000000000000000000, 1.000000000000000000, -0.000000000000000000 ) ) ;
#12706=EDGE_CURVE ( 'NONE', #7684, #8003, #10817, .T. ) ;
#12715=ADVANCED_FACE ( 'NONE', ( #13101 ), #9363, .F. ) ;
#12722=CARTESIAN_POINT ( 'NONE',  ( -20.00000000000000355, 312.0000000000000568, -2.499999999999998668 ) ) ;
#12728=DIRECTION ( 'NONE',  ( 1.000000000000000000, 0.000000000000000000, 0.000000000000000000 ) ) ;
#12732=CIRCLE ( 'NONE', #6649, 88.87749532708107836 ) ;
#12754=UNCERTAINTY_MEASURE_WITH_UNIT (LENGTH_MEASURE( 1.000000000000000082E-05 ), #15017, 'distance_accuracy_value', 'NONE');
#12758=CARTESIAN_POINT ( 'NONE',  ( 29.01527194596313564, 282.0655843567844272, -11.51527194596550530 ) ) ;
#12762=CARTESIAN_POINT ( 'NONE',  ( -25.00000000000000355, 287.0000000000000568, 2.500000000000001332 ) ) ;
#12774=CARTESIAN_POINT ( 'NONE',  ( 20.00000000000000000, 307.0000000000000568, -2.499999999999999556 ) ) ;
#12791=DIRECTION ( 'NONE',  ( -2.312964634635742464E-16, -0.000000000000000000, 1.000000000000000000 ) ) ;
#12812=CIRCLE ( 'NONE', #586, 45.00000000000000711 ) ;
#12818=EDGE_CURVE ( 'NONE', #13297, #11113, #3077, .T. ) ;
#12819=CARTESIAN_POINT ( 'NONE',  ( 30.00000000000000355, 282.0000000000000000, -12.50000000000000000 ) ) ;
#12835=CARTESIAN_POINT ( 'NONE',  ( 24.86904120090366277, 286.8604097559505703, -7.369041200904232092 ) ) ;
#12837=PLANE ( 'NONE',  #12324 ) ;
#12852=EDGE_LOOP ( 'NONE', ( #4642, #11427, #10895, #4917 ) ) ;
#12863=CARTESIAN_POINT ( 'NONE',  ( 0.000000000000000000, 267.0000000000000000, 0.000000000000000000 ) ) ;
#12872=EDGE_LOOP ( 'NONE', ( #3814, #9199, #7405, #11584 ) ) ;
#12886=VECTOR ( 'NONE', #4155, 1000.000000000000000 ) ;
#12897=VECTOR ( 'NONE', #11234, 1000.000000000000000 ) ;
#12917=ORIENTED_EDGE ( 'NONE', *, *, #14334, .T. ) ;
#12924=EDGE_CURVE ( 'NONE', #4712, #7684, #8024, .T. ) ;
#12929=CARTESIAN_POINT ( 'NONE',  ( -24.98849325795416121, 282.6608420050619088, 9.994246628976299007 ) ) ;
#12993=CARTESIAN_POINT ( 'NONE',  ( -20.00000000000000355, 287.0000000000000568, -7.499999999999999112 ) ) ;
#12998=CARTESIAN_POINT ( 'NONE',  ( -20.00000000000114042, 286.6727470533917312, -7.500000000000000888 ) ) ;
#13002=CARTESIAN_POINT ( 'NONE',  ( 29.34549410641264444, 282.0000000000000000, -12.17274705320872741 ) ) ;
#13006=CARTESIAN_POINT ( 'NONE',  ( 27.49424662897629545, 282.6608420050619088, 7.488493257954154991 ) ) ;
#13007=CARTESIAN_POINT ( 'NONE',  ( -30.00000000000000711, 282.0000000000000000, 12.50000000000000000 ) ) ;
#13010=CYLINDRICAL_SURFACE ( 'NONE', #8114, 79.49773270518484480 ) ;
#13024=DIRECTION ( 'NONE',  ( 0.000000000000000000, 0.000000000000000000, -1.000000000000000000 ) ) ;
#13084=CARTESIAN_POINT ( 'NONE',  ( 25.03223043949678939, 286.3455096218834797, 2.564460878999445193 ) ) ;
#13085=CARTESIAN_POINT ( 'NONE',  ( -24.81239020281865137, 286.7275190727449967, 7.312390202818650486 ) ) ;
#13099=AXIS2_PLACEMENT_3D ( 'NONE', #14116, #1572, #15370 ) ;
#13101=FACE_OUTER_BOUND ( 'NONE', #9218, .T. ) ;
#13164=CARTESIAN_POINT ( 'NONE',  ( 30.00000000000000355, 282.0000000000000000, 12.50000000000000178 ) ) ;
#13166=CARTESIAN_POINT ( 'NONE',  ( -21.32168401022832782, 284.4942466288906076, 8.160842005119160802 ) ) ;
#13181=ORIENTED_EDGE ( 'NONE', *, *, #10077, .F. ) ;
#13217=EDGE_LOOP ( 'NONE', ( #14340, #12292, #8605, #9572 ) ) ;
#13220=ORIENTED_EDGE ( 'NONE', *, *, #8988, .T. ) ;
#13231=APPLICATION_CONTEXT ( 'automotive_design' ) ;
#13232=DIRECTION ( 'NONE',  ( -1.000000000000000000, 6.938893903907222461E-16, 0.000000000000000000 ) ) ;
#13247=CARTESIAN_POINT ( 'NONE',  ( 29.50911996093861234, 282.0000000000000000, 12.00911996093781653 ) ) ;
#13248=CARTESIAN_POINT ( 'NONE',  ( -29.50911996093452672, 282.0000000000000000, 12.00911996094094292 ) ) ;
#13290=DIRECTION ( 'NONE',  ( 0.000000000000000000, 0.000000000000000000, 1.000000000000000000 ) ) ;
#13292=EDGE_LOOP ( 'NONE', ( #13503, #9177, #5682 ) ) ;
#13297=VERTEX_POINT ( 'NONE', #14379 ) ;
#13323=CARTESIAN_POINT ( 'NONE',  ( 25.56848793686308596, 282.5058351977237407, 10.28424396843140620 ) ) ;
#13353=AXIS2_PLACEMENT_3D ( 'NONE', #16064, #9669, #7353 ) ;
#13359=CARTESIAN_POINT ( 'NONE',  ( 0.000000000000000000, 279.6527036446661327, 0.000000000000000000 ) ) ;
#13408=ADVANCED_FACE ( 'NONE', ( #4508 ), #15552, .T. ) ;
#13429=CIRCLE ( 'NONE', #11103, 79.49773270518484480 ) ;
#13439=ORIENTED_EDGE ( 'NONE', *, *, #14107, .F. ) ;
#13456=CARTESIAN_POINT ( 'NONE',  ( 20.00000000000000000, 312.0000000000000568, 4.625929269271485322E-15 ) ) ;
#13460=VERTEX_POINT ( 'NONE', #13468 ) ;
#13468=CARTESIAN_POINT ( 'NONE',  ( 19.99999999999999289, 287.0000000000000568, -7.500000000000000000 ) ) ;
#13472=ADVANCED_FACE ( 'NONE', ( #3580 ), #16041, .F. ) ;
#13503=ORIENTED_EDGE ( 'NONE', *, *, #16408, .F. ) ;
#13514=CARTESIAN_POINT ( 'NONE',  ( -27.49424662897630256, 282.6608420050619088, -7.488493257954155879 ) ) ;
#13515=VERTEX_POINT ( 'NONE', #16291 ) ;
#13519=VERTEX_POINT ( 'NONE', #12144 ) ;
#13539=ORIENTED_EDGE ( 'NONE', *, *, #2520, .T. ) ;
#13598=AXIS2_PLACEMENT_3D ( 'NONE', #10572, #15627, #7900 ) ;
#13614=ADVANCED_FACE ( 'NONE', ( #1486 ), #8805, .T. ) ;
#13617=VERTEX_POINT ( 'NONE', #11639 ) ;
#13618=ORIENTED_EDGE ( 'NONE', *, *, #11432, .F. ) ;
#13622=ORIENTED_EDGE ( 'NONE', *, *, #10419, .T. ) ;
#13627=FACE_OUTER_BOUND ( 'NONE', #13217, .T. ) ;
#13637=AXIS2_PLACEMENT_3D ( 'NONE', #2909, #7812, #9392 ) ;
#13650=EDGE_CURVE ( 'NONE', #81, #15703, #4979, .T. ) ;
#13659=EDGE_LOOP ( 'NONE', ( #14843, #11627, #10154 ) ) ;
#13703=AXIS2_PLACEMENT_3D ( 'NONE', #7310, #9717, #14770 ) ;
#13707=ORIENTED_EDGE ( 'NONE', *, *, #16030, .F. ) ;
#13713=CARTESIAN_POINT ( 'NONE',  ( -20.00000000000000355, 307.0000000000000568, -2.499999999999998668 ) ) ;
#13720=FACE_OUTER_BOUND ( 'NONE', #4660, .T. ) ;
#13760=CARTESIAN_POINT ( 'NONE',  ( -29.01527194596337011, 282.0655843567852799, -11.51527194596495107 ) ) ;
#13778=ORIENTED_EDGE ( 'NONE', *, *, #7162, .T. ) ;
#13790=DIRECTION ( 'NONE',  ( -1.000000000000000000, 0.000000000000000000, -1.734723475976807094E-17 ) ) ;
#13793=DIRECTION ( 'NONE',  ( 0.000000000000000000, 0.000000000000000000, -1.000000000000000000 ) ) ;
#13826=VERTEX_POINT ( 'NONE', #10881 ) ;
#13839=CARTESIAN_POINT ( 'NONE',  ( -25.75618375337248622, 283.9316295015380547, -8.256183753375490042 ) ) ;
#13851=LINE ( 'NONE', #16353, #3709 ) ;
#13853=SURFACE_STYLE_FILL_AREA ( #6313 ) ;
#13865=LINE ( 'NONE', #7561, #2244 ) ;
#13878=CYLINDRICAL_SURFACE ( 'NONE', #1763, 5.000000000000000888 ) ;
#13927=DIRECTION ( 'NONE',  ( 0.000000000000000000, 1.000000000000000000, -0.000000000000000000 ) ) ;
#13933=( NAMED_UNIT ( * ) SI_UNIT ( $, .STERADIAN. ) SOLID_ANGLE_UNIT ( ) );
#13953=DIRECTION ( 'NONE',  ( 0.000000000000000000, 0.000000000000000000, 1.000000000000000000 ) ) ;
#13959=LINE ( 'NONE', #7656, #13991 ) ;
#13966=AXIS2_PLACEMENT_3D ( 'NONE', #14896, #14811, #676 ) ;
#13991=VECTOR ( 'NONE', #1322, 1000.000000000000000 ) ;
#13999=SPHERICAL_SURFACE ( 'NONE', #2001, 5.000000000000000000 ) ;
#14001=DIRECTION ( 'NONE',  ( -1.000000000000000000, 0.000000000000000000, 1.734723475976807094E-17 ) ) ;
#14008=EDGE_CURVE ( 'NONE', #6897, #13826, #16100, .T. ) ;
#14013=LINE ( 'NONE', #8704, #9531 ) ;
#14019=SURFACE_STYLE_USAGE ( .BOTH. , #8710 ) ;
#14021=AXIS2_PLACEMENT_3D ( 'NONE', #3504, #7328, #9577 ) ;
#14030=ORIENTED_EDGE ( 'NONE', *, *, #10995, .F. ) ;
#14031=ORIENTED_EDGE ( 'NONE', *, *, #2024, .F. ) ;
#14062=CARTESIAN_POINT ( 'NONE',  ( 0.000000000000000000, 272.0000000000000000, 89.49773270518483059 ) ) ;
#14069=ORIENTED_EDGE ( 'NONE', *, *, #3093, .T. ) ;
#14074=CARTESIAN_POINT ( 'NONE',  ( 26.23306594128726843, 283.6958662468472880, -4.966131882590523183 ) ) ;
#14078=DIRECTION ( 'NONE',  ( 0.000000000000000000, 0.000000000000000000, 1.000000000000000000 ) ) ;
#14088=ORIENTED_EDGE ( 'NONE', *, *, #11387, .F. ) ;
#14091=DIRECTION ( 'NONE',  ( -2.312964634635742464E-16, -0.000000000000000000, 1.000000000000000000 ) ) ;
#14095=ADVANCED_FACE ( 'NONE', ( #13720 ), #13878, .T. ) ;
#14101=DIRECTION ( 'NONE',  ( -0.000000000000000000, -1.000000000000000000, -0.000000000000000000 ) ) ;
#14103=ORIENTED_EDGE ( 'NONE', *, *, #3363, .T. ) ;
#14107=EDGE_CURVE ( 'NONE', #4375, #10042, #2413, .T. ) ;
#14116=CARTESIAN_POINT ( 'NONE',  ( 0.000000000000000000, 267.0000000000000000, 0.000000000000000000 ) ) ;
#14124=LINE ( 'NONE', #4252, #5921 ) ;
#14128=ORIENTED_EDGE ( 'NONE', *, *, #2183, .F. ) ;
#14154=CARTESIAN_POINT ( 'NONE',  ( 27.40717431545391491, 282.1599167565164521, -11.20358715772642810 ) ) ;
#14174=EDGE_CURVE ( 'NONE', #7011, #13297, #242, .T. ) ;
#14185=CARTESIAN_POINT ( 'NONE',  ( 19.99999999999999289, 307.0000000000000568, 2.500000000000002220 ) ) ;
#14203=DIRECTION ( 'NONE',  ( 0.000000000000000000, 0.000000000000000000, 1.000000000000000000 ) ) ;
#14213=ADVANCED_FACE ( 'NONE', ( #9071 ), #5508, .T. ) ;
#14219=( BOUNDED_CURVE ( )  B_SPLINE_CURVE ( 3, ( #11468, #1149, #15120, #8979 ),
 .UNSPECIFIED., .F., .F. ) 
 B_SPLINE_CURVE_WITH_KNOTS ( ( 4, 4 ),
 ( 0.000000000000000000, 1.570796326794896780 ),
 .UNSPECIFIED. ) 
 CURVE ( )  GEOMETRIC_REPRESENTATION_ITEM ( )  RATIONAL_B_SPLINE_CURVE ( ( 1.000000000000000000, 0.8047378541243649375, 0.8047378541243649375, 1.000000000000000000 ) ) 
 REPRESENTATION_ITEM ( '' )  );
#14221=DIRECTION ( 'NONE',  ( -1.000000000000000000, 0.000000000000000000, 0.000000000000000000 ) ) ;
#14224=EDGE_CURVE ( 'NONE', #8209, #5006, #14124, .T. ) ;
#14225=DIRECTION ( 'NONE',  ( 0.000000000000000000, -0.000000000000000000, 1.000000000000000000 ) ) ;
#14231=AXIS2_PLACEMENT_3D ( 'NONE', #8334, #14091, #2790 ) ;
#14235=ORIENTED_EDGE ( 'NONE', *, *, #14334, .F. ) ;
#14239=CARTESIAN_POINT ( 'NONE',  ( 22.46613188258983485, 283.6958662468469470, -8.733065941287611267 ) ) ;
#14242=AXIS2_PLACEMENT_3D ( 'NONE', #10337, #8832, #4018 ) ;
#14246=CARTESIAN_POINT ( 'NONE',  ( 26.95005104082769520, 283.0244618719127629, 6.400102081653809449 ) ) ;
#14259=ORIENTED_EDGE ( 'NONE', *, *, #9388, .T. ) ;
#14262=CARTESIAN_POINT ( 'NONE',  ( 0.000000000000000000, 273.6527036446661896, 0.000000000000000000 ) ) ;
#14293=ORIENTED_EDGE ( 'NONE', *, *, #15309, .F. ) ;
#14327=CARTESIAN_POINT ( 'NONE',  ( -24.76951992798375102, 286.3033656649002410, 7.269519927983750129 ) ) ;
#14334=EDGE_CURVE ( 'NONE', #6698, #11113, #9396, .T. ) ;
#14340=ORIENTED_EDGE ( 'NONE', *, *, #14224, .F. ) ;
#14366=DIRECTION ( 'NONE',  ( 0.000000000000000000, -1.000000000000000000, 0.000000000000000000 ) ) ;
#14379=CARTESIAN_POINT ( 'NONE',  ( 25.00000000000000000, 307.0000000000000568, -2.499999999999997780 ) ) ;
#14380=DIRECTION ( 'NONE',  ( 1.224646799147349509E-16, 0.000000000000000000, -1.000000000000000000 ) ) ;
#14395=CARTESIAN_POINT ( 'NONE',  ( 1.112556234935474772E-14, 279.6527036446661327, -90.84711083310548929 ) ) ;
#14397=CARTESIAN_POINT ( 'NONE',  ( 29.01527194596310721, 282.0655843567844272, 11.51527194596232206 ) ) ;
#14398=CARTESIAN_POINT ( 'NONE',  ( -20.00000000000114042, 286.6727470533917312, 7.500000000000002665 ) ) ;
#14403=CIRCLE ( 'NONE', #2998, 5.000000000000004441 ) ;
#14444=EDGE_LOOP ( 'NONE', ( #10402, #9048, #13618, #7400 ) ) ;
#14456=VECTOR ( 'NONE', #13927, 1000.000000000000000 ) ;
#14473=CARTESIAN_POINT ( 'NONE',  ( 23.39173249367787122, 283.2330659412879186, 9.195866246846582825 ) ) ;
#14474=CARTESIAN_POINT ( 'NONE',  ( -21.01167039530930936, 284.7842439685843487, 8.005835197660418956 ) ) ;
#14491=ORIENTED_EDGE ( 'NONE', *, *, #14773, .T. ) ;
#14505=AXIS2_PLACEMENT_3D ( 'NONE', #5061, #2447, #3713 ) ;
#14530=ORIENTED_EDGE ( 'NONE', *, *, #16267, .T. ) ;
#14533=EDGE_LOOP ( 'NONE', ( #4333, #3733, #13220, #3034 ) ) ;
#14541=CARTESIAN_POINT ( 'NONE',  ( -30.00000000000000711, 282.0000000000000000, -12.49999999999999822 ) ) ;
#14542=DIRECTION ( 'NONE',  ( 0.000000000000000000, 1.000000000000000000, 0.000000000000000000 ) ) ;
#14554=EDGE_LOOP ( 'NONE', ( #14491, #11223, #3553, #14103 ) ) ;
#14586=DIRECTION ( 'NONE',  ( 0.000000000000000000, 1.000000000000000000, 0.000000000000000000 ) ) ;
#14590=ORIENTED_EDGE ( 'NONE', *, *, #4797, .T. ) ;
#14672=EDGE_CURVE ( 'NONE', #7881, #11148, #2181, .T. ) ;
#14675=DIRECTION ( 'NONE',  ( -0.000000000000000000, -1.000000000000000000, -0.000000000000000000 ) ) ;
#14702=DIRECTION ( 'NONE',  ( 0.000000000000000000, 0.000000000000000000, 1.000000000000000000 ) ) ;
#14706=CARTESIAN_POINT ( 'NONE',  ( -25.00000000000000355, 307.0000000000000568, -2.499999999999998668 ) ) ;
#14735=VERTEX_POINT ( 'NONE', #7639 ) ;
#14751=CARTESIAN_POINT ( 'NONE',  ( -27.40717431545314042, 282.1599167565163384, -11.20358715772689351 ) ) ;
#14759=ORIENTED_EDGE ( 'NONE', *, *, #4797, .F. ) ;
#14760=ORIENTED_EDGE ( 'NONE', *, *, #16030, .T. ) ;
#14770=DIRECTION ( 'NONE',  ( 0.000000000000000000, 0.000000000000000000, 1.000000000000000000 ) ) ;
#14773=EDGE_CURVE ( 'NONE', #10689, #10428, #2559, .T. ) ;
#14774=DIRECTION ( 'NONE',  ( 2.312964634635742464E-16, 0.000000000000000000, -1.000000000000000000 ) ) ;
#14779=ORIENTED_EDGE ( 'NONE', *, *, #11697, .F. ) ;
#14801=CARTESIAN_POINT ( 'NONE',  ( -20.00000000000000355, 307.0000000000000568, 7.500000000000001776 ) ) ;
#14802=CIRCLE ( 'NONE', #11116, 5.000000000000000000 ) ;
#14803=EDGE_LOOP ( 'NONE', ( #14031, #7945, #11015, #98 ) ) ;
#14807=EDGE_CURVE ( 'NONE', #8209, #4375, #12812, .T. ) ;
#14811=DIRECTION ( 'NONE',  ( 0.000000000000000000, -1.000000000000000000, 0.000000000000000000 ) ) ;
#14827=ORIENTED_EDGE ( 'NONE', *, *, #3093, .F. ) ;
#14832=ADVANCED_FACE ( 'NONE', ( #9541 ), #4599, .T. ) ;
#14838=ORIENTED_EDGE ( 'NONE', *, *, #15040, .T. ) ;
#14843=ORIENTED_EDGE ( 'NONE', *, *, #512, .F. ) ;
#14848=( BOUNDED_SURFACE ( )  B_SPLINE_SURFACE ( 3, 2, ( 
 ( #9018, #3863, #11671 ),
 ( #13002, #12680, #2860 ),
 ( #5208, #12758, #11506 ),
 ( #14154, #103, #5131 ),
 ( #15484, #5375, #5297 ),
 ( #7929, #9179, #10266 ),
 ( #190, #2770, #10429 ),
 ( #15326, #2612, #270 ),
 ( #1355, #3945, #7688 ),
 ( #14239, #10345, #14074 ),
 ( #11591, #4108, #1528 ),
 ( #1606, #16419, #2689 ),
 ( #25, #11433, #1277 ),
 ( #15409, #4026, #6528 ),
 ( #7764, #12835, #7845 ),
 ( #3783, #11354, #6367 ),
 ( #5054, #8933, #9096 ),
 ( #10105, #6447, #10184 ) ),
 .UNSPECIFIED., .F., .F., .F. ) 
 B_SPLINE_SURFACE_WITH_KNOTS ( ( 4, 2, 2, 2, 2, 2, 2, 2, 4 ),
 ( 3, 3 ),
 ( 4.712388980384689674, 4.908738521234051966, 5.105088062083414258, 5.301437602932775661, 5.497787143782137953, 5.694136684631500245, 5.890486225480861648, 6.086835766330223940, 6.283185307179586232 ),
 ( 0.000000000000000000, 1.000000000000000000 ),
 .UNSPECIFIED. ) 
 GEOMETRIC_REPRESENTATION_ITEM ( )  RATIONAL_B_SPLINE_SURFACE ( (
 ( 1.000000000000000000, 1.000000000000000000, 1.000000000000000000),
 ( 1.000000000000000000, 1.000000000000000000, 1.000000000000000000),
 ( 1.000000000000000000, 0.9967613244521382754, 1.000000000000000000),
 ( 1.000000000000000000, 0.9841171504956023330, 1.000000000000000000),
 ( 1.000000000000000000, 0.9747108043452729076, 1.000000000000000000),
 ( 1.000000000000000000, 0.9506740354170398755, 1.000000000000000000),
 ( 1.000000000000000000, 0.9360421842396995373, 1.000000000000000000),
 ( 1.000000000000000000, 0.9031650994466967619, 1.000000000000000000),
 ( 1.000000000000000000, 0.8849191470849313568, 1.000000000000000000),
 ( 1.000000000000000000, 0.8471316604839480569, 1.000000000000000000),
 ( 1.000000000000000000, 0.8275942695270729343, 1.000000000000000000),
 ( 1.000000000000000000, 0.7902180087162717914, 1.000000000000000000),
 ( 1.000000000000000000, 0.7723968217384142854, 1.000000000000000000),
 ( 1.000000000000000000, 0.7418334179587914301, 1.000000000000000000),
 ( 1.000000000000000000, 0.7291288939600963914, 1.000000000000000000),
 ( 1.000000000000000000, 0.7117460025832214043, 1.000000000000000000),
 ( 1.000000000000000000, 0.7070717283367429218, 1.000000000000000000),
 ( 1.000000000000000000, 0.7071067811865474617, 1.000000000000000000) ) ) 
 REPRESENTATION_ITEM ( '' )  SURFACE ( )  );
#14873=CARTESIAN_POINT ( 'NONE',  ( -30.00000000000000711, 282.0000000000000000, 12.50000000000000000 ) ) ;
#14896=CARTESIAN_POINT ( 'NONE',  ( 0.000000000000000000, 267.0000000000000000, 0.000000000000000000 ) ) ;
#14927=FACE_OUTER_BOUND ( 'NONE', #14533, .T. ) ;
#14929=LINE ( 'NONE', #2462, #3685 ) ;
#14936=( LENGTH_UNIT ( ) NAMED_UNIT ( * ) SI_UNIT ( .MILLI., .METRE. ) );
#14940=ADVANCED_FACE ( 'NONE', ( #16184 ), #1603, .T. ) ;
#14960=CARTESIAN_POINT ( 'NONE',  ( -24.14213562373095101, 282.0000000000000000, -9.571067811865473729 ) ) ;
#14969=ORIENTED_EDGE ( 'NONE', *, *, #4986, .F. ) ;
#14983=DIRECTION ( 'NONE',  ( 1.000000000000000000, 0.000000000000000000, 0.000000000000000000 ) ) ;
#14997=CIRCLE ( 'NONE', #11299, 87.81953344283027718 ) ;
#15002=CARTESIAN_POINT ( 'NONE',  ( -22.04892374372078834, 283.9500510409131948, -8.524461871855592676 ) ) ;
#15005=ORIENTED_EDGE ( 'NONE', *, *, #6524, .F. ) ;
#15010=CYLINDRICAL_SURFACE ( 'NONE', #10561, 5.000000000000000000 ) ;
#15017=( LENGTH_UNIT ( ) NAMED_UNIT ( * ) SI_UNIT ( .MILLI., .METRE. ) );
#15040=EDGE_CURVE ( 'NONE', #12589, #11148, #11823, .T. ) ;
#15059=DIRECTION ( 'NONE',  ( 0.000000000000000000, -1.000000000000000000, 0.000000000000000000 ) ) ;
#15065=DIRECTION ( 'NONE',  ( 0.000000000000000000, 0.000000000000000000, 1.000000000000000000 ) ) ;
#15081=DIRECTION ( 'NONE',  ( 0.000000000000000000, -0.000000000000000000, -1.000000000000000000 ) ) ;
#15083=CARTESIAN_POINT ( 'NONE',  ( 0.000000000000000000, 262.0000000000000000, 0.000000000000000000 ) ) ;
#15102=( NAMED_UNIT ( * ) PLANE_ANGLE_UNIT ( ) SI_UNIT ( $, .RADIAN. ) );
#15104=( NAMED_UNIT ( * ) PLANE_ANGLE_UNIT ( ) SI_UNIT ( $, .RADIAN. ) );
#15113=ORIENTED_EDGE ( 'NONE', *, *, #4920, .F. ) ;
#15114=CARTESIAN_POINT ( 'NONE',  ( 0.000000000000000000, 262.0000000000000000, 0.000000000000000000 ) ) ;
#15120=CARTESIAN_POINT ( 'NONE',  ( 27.07106781186547551, 282.0000000000000000, 6.642135623730952787 ) ) ;
#15131=ORIENTED_EDGE ( 'NONE', *, *, #15522, .F. ) ;
#15163=CARTESIAN_POINT ( 'NONE',  ( -25.00000000000000355, 287.0000000000000568, -7.499999999999999112 ) ) ;
#15174=CARTESIAN_POINT ( 'NONE',  ( -20.00000000000000355, 312.0000000000000568, 0.000000000000000000 ) ) ;
#15188=ORIENTED_EDGE ( 'NONE', *, *, #8988, .F. ) ;
#15207=ORIENTED_EDGE ( 'NONE', *, *, #15040, .F. ) ;
#15229=APPLICATION_CONTEXT ( 'automotive_design' ) ;
#15231=UNCERTAINTY_MEASURE_WITH_UNIT (LENGTH_MEASURE( 1.000000000000000082E-05 ), #14936, 'distance_accuracy_value', 'NONE');
#15233=ORIENTED_EDGE ( 'NONE', *, *, #10477, .F. ) ;
#15242=DIRECTION ( 'NONE',  ( 0.000000000000000000, 1.000000000000000000, 0.000000000000000000 ) ) ;
#15260=FACE_OUTER_BOUND ( 'NONE', #2378, .T. ) ;
#15263=ADVANCED_FACE ( 'NONE', ( #1609 ), #6092, .T. ) ;
#15265=DIRECTION ( 'NONE',  ( 0.000000000000000000, 0.000000000000000000, -1.000000000000000000 ) ) ;
#15268=PRODUCT ( 'lid', 'lid', '', ( #464 ) ) ;
#15285=AXIS2_PLACEMENT_3D ( 'NONE', #3126, #3602, #7265 ) ;
#15287=PRODUCT_DEFINITION_FORMATION_WITH_SPECIFIED_SOURCE ( 'ANY', '', #15268, .NOT_KNOWN. ) ;
#15297=AXIS2_PLACEMENT_3D ( 'NONE', #15083, #11437, #2693 ) ;
#15309=EDGE_CURVE ( 'NONE', #11113, #8227, #675, .T. ) ;
#15322=AXIS2_PLACEMENT_3D ( 'NONE', #2932, #5603, #2851 ) ;
#15323=EDGE_CURVE ( 'NONE', #5006, #10042, #11248, .T. ) ;
#15325=ORIENTED_EDGE ( 'NONE', *, *, #12924, .F. ) ;
#15326=CARTESIAN_POINT ( 'NONE',  ( 23.90010208165381300, 283.0244618719127629, -9.450051040827696980 ) ) ;
#15330=PLANE ( 'NONE',  #15297 ) ;
#15352=SHAPE_DEFINITION_REPRESENTATION ( #9190, #329 ) ;
#15370=DIRECTION ( 'NONE',  ( 0.000000000000000000, 0.000000000000000000, -1.000000000000000000 ) ) ;
#15378=ORIENTED_EDGE ( 'NONE', *, *, #5864, .F. ) ;
#15384=CARTESIAN_POINT ( 'NONE',  ( 0.000000000000000000, 274.0000000000000000, 87.81953344283027718 ) ) ;
#15403=ORIENTED_EDGE ( 'NONE', *, *, #4586, .F. ) ;
#15409=CARTESIAN_POINT ( 'NONE',  ( 20.51073895446738504, 285.3889217077638705, -7.755369477227150199 ) ) ;
#15424=DIRECTION ( 'NONE',  ( -2.312964634635742464E-16, 0.000000000000000000, 1.000000000000000000 ) ) ;
#15433=CYLINDRICAL_SURFACE ( 'NONE', #9683, 45.00000000000000711 ) ;
#15437=EDGE_CURVE ( 'NONE', #11113, #12621, #14403, .T. ) ;
#15458=ORIENTED_EDGE ( 'NONE', *, *, #4378, .T. ) ;
#15465=VECTOR ( 'NONE', #2915, 1000.000000000000000 ) ;
#15471=CARTESIAN_POINT ( 'NONE',  ( -25.00000000000000355, 312.0000000000000568, -2.499999999999998668 ) ) ;
#15475=DIRECTION ( 'NONE',  ( 0.000000000000000000, 1.000000000000000000, 0.000000000000000000 ) ) ;
#15484=CARTESIAN_POINT ( 'NONE',  ( 26.77784341583361183, 282.2553694771637538, -10.88892170791706171 ) ) ;
#15488=CARTESIAN_POINT ( 'NONE',  ( 29.67274705320743422, 282.0000000000000000, 11.84549410641326617 ) ) ;
#15522=EDGE_CURVE ( 'NONE', #7238, #12589, #2577, .T. ) ;
#15534=VECTOR ( 'NONE', #9860, 1000.000000000000000 ) ;
#15552=CYLINDRICAL_SURFACE ( 'NONE', #9735, 5.000000000000000000 ) ;
#15577=LINE ( 'NONE', #7847, #4646 ) ;
#15579=CARTESIAN_POINT ( 'NONE',  ( 30.00000000000000000, 282.0000000000000000, 12.50000000000000178 ) ) ;
#15581=CARTESIAN_POINT ( 'NONE',  ( -25.75618375337248978, 283.9316295015381115, 8.256183753373989020 ) ) ;
#15584=FACE_OUTER_BOUND ( 'NONE', #1004, .T. ) ;
#15589=CONICAL_SURFACE ( 'NONE', #1785, 89.49773270518483059, 0.1745329251994333364 ) ;
#15627=DIRECTION ( 'NONE',  ( 0.000000000000000000, -1.000000000000000000, 0.000000000000000000 ) ) ;
#15659=CARTESIAN_POINT ( 'NONE',  ( 27.40717431545390781, 282.1599167565162816, 11.20358715772719371 ) ) ;
#15662=CARTESIAN_POINT ( 'NONE',  ( -28.70358715772690061, 282.1599167565163384, 9.907174315453929125 ) ) ;
#15703=VERTEX_POINT ( 'NONE', #8556 ) ;
#15715=DIRECTION ( 'NONE',  ( -0.000000000000000000, -1.000000000000000000, 0.000000000000000000 ) ) ;
#15730=CARTESIAN_POINT ( 'NONE',  ( 24.76951992798502999, 286.3033656649012642, 7.269519927984441132 ) ) ;
#15731=CARTESIAN_POINT ( 'NONE',  ( -26.78441608355137049, 282.9883952696293932, 9.284416083550581789 ) ) ;
#15734=DIRECTION ( 'NONE',  ( 1.734723475976807094E-17, 0.000000000000000000, 1.000000000000000000 ) ) ;
#15776=ADVANCED_FACE ( 'NONE', ( #13627 ), #11158, .F. ) ;
#15786=EDGE_LOOP ( 'NONE', ( #4181, #14259 ) ) ;
#15808=AXIS2_PLACEMENT_3D ( 'NONE', #6289, #7522, #14078 ) ;
#15812=AXIS2_PLACEMENT_3D ( 'NONE', #2158, #11073, #8560 ) ;
#15817=CARTESIAN_POINT ( 'NONE',  ( -24.93825083352641769, 285.3724546740604637, 7.438250833527376926 ) ) ;
#15834=CIRCLE ( 'NONE', #15322, 5.000000000000000000 ) ;
#15836=ORIENTED_EDGE ( 'NONE', *, *, #2183, .T. ) ;
#15846=ADVANCED_FACE ( 'NONE', ( #3503 ), #12146, .F. ) ;
#15857=ORIENTED_EDGE ( 'NONE', *, *, #12924, .T. ) ;
#15864=ADVANCED_FACE ( 'NONE', ( #4766 ), #16287, .T. ) ;
#15868=DIRECTION ( 'NONE',  ( 1.000000000000000000, -0.000000000000000000, 1.224646799147353207E-16 ) ) ;
#15886=CARTESIAN_POINT ( 'NONE',  ( 0.000000000000000000, 279.6527036446661327, 0.000000000000000000 ) ) ;
#15962=CARTESIAN_POINT ( 'NONE',  ( -25.00000000000000355, 312.0000000000000568, 7.500000000000001776 ) ) ;
#15971=ADVANCED_FACE ( 'NONE', ( #6332 ), #872, .T. ) ;
#15981=CARTESIAN_POINT ( 'NONE',  ( 20.00000000000113332, 286.6727470533786573, 7.500000000000000888 ) ) ;
#15995=EDGE_LOOP ( 'NONE', ( #7539, #14293, #52, #3919 ) ) ;
#16003=FACE_OUTER_BOUND ( 'NONE', #9855, .T. ) ;
#16010=ORIENTED_EDGE ( 'NONE', *, *, #11387, .T. ) ;
#16030=EDGE_CURVE ( 'NONE', #6698, #11148, #8326, .T. ) ;
#16041=PLANE ( 'NONE',  #6813 ) ;
#16044=FACE_OUTER_BOUND ( 'NONE', #3121, .T. ) ;
#16064=CARTESIAN_POINT ( 'NONE',  ( 0.000000000000000000, 262.0000000000000000, 0.000000000000000000 ) ) ;
#16086=AXIS2_PLACEMENT_3D ( 'NONE', #13713, #10372, #12481 ) ;
#16095=EDGE_CURVE ( 'NONE', #4375, #8209, #5947, .T. ) ;
#16098=CARTESIAN_POINT ( 'NONE',  ( -28.38892170791837799, 282.2553694771631854, -9.277843415833588736 ) ) ;
#16100=CIRCLE ( 'NONE', #13703, 2.000000000000001776 ) ;
#16105=ORIENTED_EDGE ( 'NONE', *, *, #6712, .T. ) ;
#16112=CIRCLE ( 'NONE', #11080, 5.000000000000000000 ) ;
#16139=DIRECTION ( 'NONE',  ( 0.000000000000000000, 0.000000000000000000, 1.000000000000000000 ) ) ;
#16156=CARTESIAN_POINT ( 'NONE',  ( 25.00000000000000000, 287.0000000000000000, 7.500000000000000888 ) ) ;
#16184=FACE_OUTER_BOUND ( 'NONE', #13292, .T. ) ;
#16187=CARTESIAN_POINT ( 'NONE',  ( 24.14213562373095101, 282.0000000000000000, -9.571067811865473729 ) ) ;
#16190=ORIENTED_EDGE ( 'NONE', *, *, #12818, .T. ) ;
#16214=CARTESIAN_POINT ( 'NONE',  ( 0.000000000000000000, 274.0000000000000000, 0.000000000000000000 ) ) ;
#16256=CARTESIAN_POINT ( 'NONE',  ( -21.01167039530930936, 284.7842439685843487, -8.005835197660415403 ) ) ;
#16267=EDGE_CURVE ( 'NONE', #8227, #12043, #10188, .T. ) ;
#16272=PRESENTATION_STYLE_ASSIGNMENT (( #1051 ) ) ;
#16287=TOROIDAL_SURFACE ( 'NONE', #1410, 87.81953344283027718, 2.000000000000000000 ) ;
#16291=CARTESIAN_POINT ( 'NONE',  ( -20.00000000000000355, 312.0000000000000568, 2.500000000000001332 ) ) ;
#16293=CARTESIAN_POINT ( 'NONE',  ( 20.00000000000000000, 307.0000000000000568, 2.500000000000002220 ) ) ;
#16295=DIRECTION ( 'NONE',  ( -0.000000000000000000, 1.000000000000000000, 0.000000000000000000 ) ) ;
#16296=CYLINDRICAL_SURFACE ( 'NONE', #2760, 40.00000000000000000 ) ;
#16334=CARTESIAN_POINT ( 'NONE',  ( 9.735664389687646693E-15, 262.0000000000000000, -79.49773270518484480 ) ) ;
#16347=CARTESIAN_POINT ( 'NONE',  ( 0.000000000000000000, 262.0000000000000000, 0.000000000000000000 ) ) ;
#16353=CARTESIAN_POINT ( 'NONE',  ( -25.00000000000000355, 307.0000000000000568, -7.499999999999999112 ) ) ;
#16357=FACE_OUTER_BOUND ( 'NONE', #15786, .T. ) ;
#16364=ORIENTED_EDGE ( 'NONE', *, *, #12618, .T. ) ;
#16375=VERTEX_POINT ( 'NONE', #7089 ) ;
#16408=EDGE_CURVE ( 'NONE', #10428, #891, #8403, .T. ) ;
#16419=CARTESIAN_POINT ( 'NONE',  ( 24.78235906513272724, 286.0218276482402189, -7.282359065131384313 ) ) ;
#16425=LINE ( 'NONE', #15163, #6309 ) ;
#16432=CARTESIAN_POINT ( 'NONE',  ( -20.06446087899944786, 286.3455096218657445, -7.532230439500316344 ) ) ;
#16451=CARTESIAN_POINT ( 'NONE',  ( 1.087539521958779419E-14, 272.0000000000000000, -87.81953344283027718 ) ) ;
ENDSEC;
END-ISO-10303-21;
